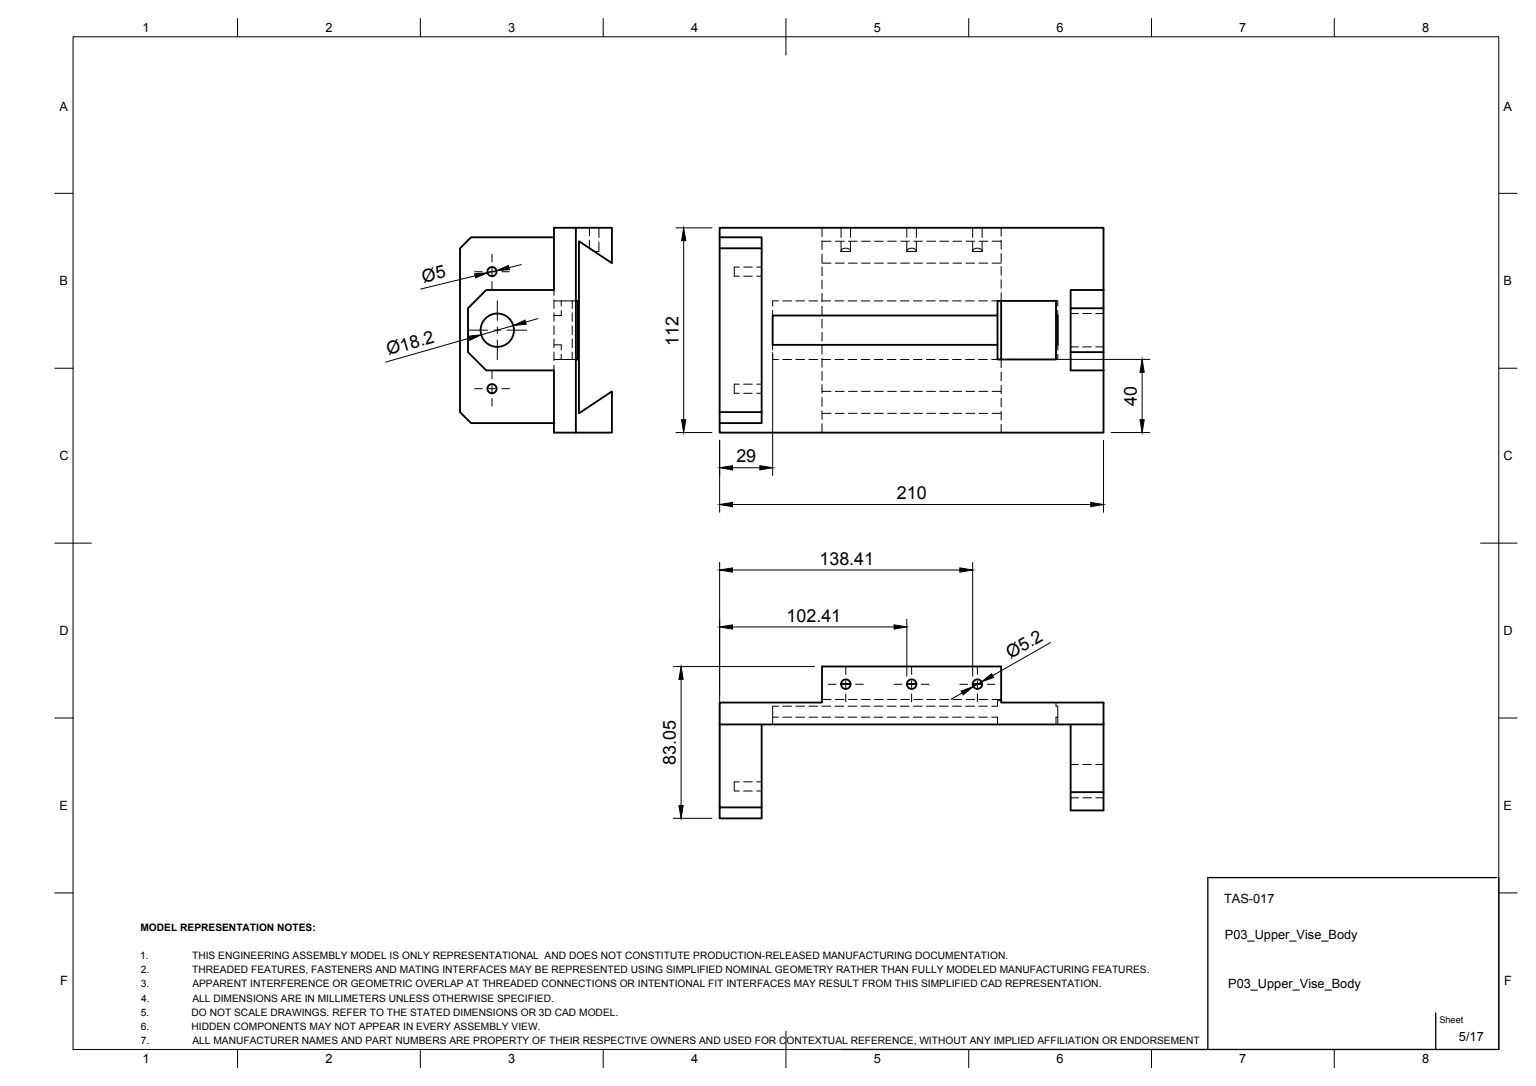
ISO-10303-21;
HEADER;
/* Generated by software containing ST-Developer
 * from STEP Tools, Inc. (www.steptools.com) 
 */

FILE_DESCRIPTION(
/* description */ ('STEP AP203'),
/* implementation_level */ '2;1');

FILE_NAME(
/* name */ 'P03_Upper_Vise_Body.step',
/* time_stamp */ '2026-11-15T15:04:01-08:00',
/* author */ (''),
/* organization */ (''),
/* preprocessor_version */ 'ST-DEVELOPER v20.2',
/* originating_system */ 'Autodesk Translation Framework v15.17.0.0',
/* authorisation */ '');

FILE_SCHEMA (('AUTOMOTIVE_DESIGN { 1 0 10303 214 3 1 1 }'));
ENDSEC;

DATA;
#10=MECHANICAL_DESIGN_GEOMETRIC_PRESENTATION_REPRESENTATION('',(#282),#16598);
#201=ELLIPSE('',#10193,3.12481110540202,2.59999999999971);
#202=ELLIPSE('',#10198,3.1248111054012,2.59999999999909);
#203=ELLIPSE('',#10203,3.12481110540162,2.59999999999945);
#206=SHAPE_REPRESENTATION_RELATIONSHIP('SRR','None',#16700,#230);
#230=ADVANCED_BREP_SHAPE_REPRESENTATION('',(#254),#16576);
#254=MANIFOLD_SOLID_BREP('Body1',#9789);
#282=STYLED_ITEM('',(#16830),#254);
#320=FACE_BOUND('',#1569,.T.);
#321=FACE_BOUND('',#1583,.T.);
#322=FACE_BOUND('',#1584,.T.);
#323=FACE_BOUND('',#1585,.T.);
#324=FACE_BOUND('',#1587,.T.);
#325=FACE_BOUND('',#1588,.T.);
#326=FACE_BOUND('',#1589,.T.);
#327=FACE_BOUND('',#1597,.T.);
#328=FACE_BOUND('',#1606,.T.);
#329=FACE_BOUND('',#1607,.T.);
#330=FACE_BOUND('',#1614,.T.);
#506=PLANE('',#10214);
#507=PLANE('',#10215);
#508=PLANE('',#10216);
#509=PLANE('',#10217);
#510=PLANE('',#10218);
#511=PLANE('',#10219);
#512=PLANE('',#10220);
#513=PLANE('',#10221);
#514=PLANE('',#10222);
#515=PLANE('',#10223);
#516=PLANE('',#10224);
#517=PLANE('',#10225);
#518=PLANE('',#10226);
#519=PLANE('',#10227);
#520=PLANE('',#10228);
#521=PLANE('',#10229);
#522=PLANE('',#10230);
#523=PLANE('',#10231);
#524=PLANE('',#10232);
#525=PLANE('',#10233);
#526=PLANE('',#10234);
#527=PLANE('',#10235);
#528=PLANE('',#10236);
#529=PLANE('',#10237);
#530=PLANE('',#10238);
#531=PLANE('',#10239);
#532=PLANE('',#10240);
#533=PLANE('',#10241);
#534=PLANE('',#10242);
#535=PLANE('',#10243);
#536=PLANE('',#10244);
#537=PLANE('',#10245);
#538=PLANE('',#10246);
#539=PLANE('',#10247);
#540=PLANE('',#10248);
#541=PLANE('',#10249);
#542=PLANE('',#10250);
#543=PLANE('',#10251);
#544=PLANE('',#10252);
#545=PLANE('',#10253);
#546=PLANE('',#10254);
#547=PLANE('',#10255);
#548=PLANE('',#10256);
#549=PLANE('',#10257);
#550=PLANE('',#10258);
#551=PLANE('',#10259);
#552=PLANE('',#10260);
#553=PLANE('',#10261);
#554=PLANE('',#10262);
#555=PLANE('',#10263);
#556=PLANE('',#10264);
#557=PLANE('',#10265);
#997=FACE_OUTER_BOUND('',#1562,.T.);
#998=FACE_OUTER_BOUND('',#1563,.T.);
#999=FACE_OUTER_BOUND('',#1564,.T.);
#1000=FACE_OUTER_BOUND('',#1565,.T.);
#1001=FACE_OUTER_BOUND('',#1566,.T.);
#1002=FACE_OUTER_BOUND('',#1567,.T.);
#1003=FACE_OUTER_BOUND('',#1568,.T.);
#1004=FACE_OUTER_BOUND('',#1570,.T.);
#1005=FACE_OUTER_BOUND('',#1571,.T.);
#1006=FACE_OUTER_BOUND('',#1572,.T.);
#1007=FACE_OUTER_BOUND('',#1573,.T.);
#1008=FACE_OUTER_BOUND('',#1574,.T.);
#1009=FACE_OUTER_BOUND('',#1575,.T.);
#1010=FACE_OUTER_BOUND('',#1576,.T.);
#1011=FACE_OUTER_BOUND('',#1577,.T.);
#1012=FACE_OUTER_BOUND('',#1578,.T.);
#1013=FACE_OUTER_BOUND('',#1579,.T.);
#1014=FACE_OUTER_BOUND('',#1580,.T.);
#1015=FACE_OUTER_BOUND('',#1581,.T.);
#1016=FACE_OUTER_BOUND('',#1582,.T.);
#1017=FACE_OUTER_BOUND('',#1586,.T.);
#1018=FACE_OUTER_BOUND('',#1590,.T.);
#1019=FACE_OUTER_BOUND('',#1591,.T.);
#1020=FACE_OUTER_BOUND('',#1592,.T.);
#1021=FACE_OUTER_BOUND('',#1593,.T.);
#1022=FACE_OUTER_BOUND('',#1594,.T.);
#1023=FACE_OUTER_BOUND('',#1595,.T.);
#1024=FACE_OUTER_BOUND('',#1596,.T.);
#1025=FACE_OUTER_BOUND('',#1598,.T.);
#1026=FACE_OUTER_BOUND('',#1599,.T.);
#1027=FACE_OUTER_BOUND('',#1600,.T.);
#1028=FACE_OUTER_BOUND('',#1601,.T.);
#1029=FACE_OUTER_BOUND('',#1602,.T.);
#1030=FACE_OUTER_BOUND('',#1603,.T.);
#1031=FACE_OUTER_BOUND('',#1604,.T.);
#1032=FACE_OUTER_BOUND('',#1605,.T.);
#1033=FACE_OUTER_BOUND('',#1608,.T.);
#1034=FACE_OUTER_BOUND('',#1609,.T.);
#1035=FACE_OUTER_BOUND('',#1610,.T.);
#1036=FACE_OUTER_BOUND('',#1611,.T.);
#1037=FACE_OUTER_BOUND('',#1612,.T.);
#1038=FACE_OUTER_BOUND('',#1613,.T.);
#1039=FACE_OUTER_BOUND('',#1615,.T.);
#1040=FACE_OUTER_BOUND('',#1616,.T.);
#1041=FACE_OUTER_BOUND('',#1617,.T.);
#1042=FACE_OUTER_BOUND('',#1618,.T.);
#1043=FACE_OUTER_BOUND('',#1619,.T.);
#1044=FACE_OUTER_BOUND('',#1620,.T.);
#1045=FACE_OUTER_BOUND('',#1621,.T.);
#1046=FACE_OUTER_BOUND('',#1622,.T.);
#1047=FACE_OUTER_BOUND('',#1623,.T.);
#1048=FACE_OUTER_BOUND('',#1624,.T.);
#1049=FACE_OUTER_BOUND('',#1625,.T.);
#1050=FACE_OUTER_BOUND('',#1626,.T.);
#1051=FACE_OUTER_BOUND('',#1627,.T.);
#1052=FACE_OUTER_BOUND('',#1628,.T.);
#1053=FACE_OUTER_BOUND('',#1629,.T.);
#1054=FACE_OUTER_BOUND('',#1630,.T.);
#1562=EDGE_LOOP('',(#7041,#7042,#7043,#7044,#7045,#7046));
#1563=EDGE_LOOP('',(#7047,#7048,#7049,#7050,#7051,#7052));
#1564=EDGE_LOOP('',(#7053,#7054,#7055,#7056,#7057,#7058));
#1565=EDGE_LOOP('',(#7059,#7060,#7061,#7062));
#1566=EDGE_LOOP('',(#7063,#7064,#7065,#7066));
#1567=EDGE_LOOP('',(#7067,#7068,#7069,#7070));
#1568=EDGE_LOOP('',(#7071,#7072,#7073,#7074,#7075,#7076,#7077,#7078,#7079,
#7080,#7081,#7082));
#1569=EDGE_LOOP('',(#7083,#7084,#7085,#7086,#7087,#7088,#7089,#7090,#7091,
#7092,#7093,#7094));
#1570=EDGE_LOOP('',(#7095,#7096,#7097,#7098,#7099,#7100,#7101,#7102,#7103,
#7104,#7105,#7106));
#1571=EDGE_LOOP('',(#7107,#7108,#7109,#7110,#7111,#7112,#7113,#7114));
#1572=EDGE_LOOP('',(#7115,#7116,#7117,#7118));
#1573=EDGE_LOOP('',(#7119,#7120,#7121,#7122));
#1574=EDGE_LOOP('',(#7123,#7124,#7125,#7126));
#1575=EDGE_LOOP('',(#7127,#7128,#7129,#7130));
#1576=EDGE_LOOP('',(#7131,#7132,#7133,#7134));
#1577=EDGE_LOOP('',(#7135,#7136,#7137,#7138));
#1578=EDGE_LOOP('',(#7139,#7140,#7141,#7142));
#1579=EDGE_LOOP('',(#7143,#7144,#7145,#7146));
#1580=EDGE_LOOP('',(#7147,#7148,#7149,#7150));
#1581=EDGE_LOOP('',(#7151,#7152,#7153,#7154));
#1582=EDGE_LOOP('',(#7155,#7156,#7157,#7158));
#1583=EDGE_LOOP('',(#7159,#7160));
#1584=EDGE_LOOP('',(#7161,#7162));
#1585=EDGE_LOOP('',(#7163,#7164));
#1586=EDGE_LOOP('',(#7165,#7166,#7167,#7168,#7169,#7170,#7171,#7172));
#1587=EDGE_LOOP('',(#7173));
#1588=EDGE_LOOP('',(#7174));
#1589=EDGE_LOOP('',(#7175));
#1590=EDGE_LOOP('',(#7176,#7177,#7178,#7179));
#1591=EDGE_LOOP('',(#7180,#7181,#7182,#7183));
#1592=EDGE_LOOP('',(#7184,#7185,#7186,#7187));
#1593=EDGE_LOOP('',(#7188,#7189,#7190,#7191));
#1594=EDGE_LOOP('',(#7192,#7193,#7194,#7195,#7196,#7197,#7198,#7199));
#1595=EDGE_LOOP('',(#7200,#7201,#7202,#7203,#7204,#7205,#7206,#7207));
#1596=EDGE_LOOP('',(#7208,#7209,#7210,#7211,#7212,#7213,#7214,#7215,#7216,
#7217));
#1597=EDGE_LOOP('',(#7218));
#1598=EDGE_LOOP('',(#7219,#7220,#7221,#7222));
#1599=EDGE_LOOP('',(#7223,#7224,#7225,#7226,#7227,#7228,#7229,#7230,#7231,
#7232));
#1600=EDGE_LOOP('',(#7233,#7234,#7235,#7236));
#1601=EDGE_LOOP('',(#7237,#7238,#7239,#7240));
#1602=EDGE_LOOP('',(#7241,#7242,#7243,#7244));
#1603=EDGE_LOOP('',(#7245,#7246,#7247,#7248));
#1604=EDGE_LOOP('',(#7249,#7250,#7251,#7252));
#1605=EDGE_LOOP('',(#7253,#7254,#7255,#7256,#7257,#7258));
#1606=EDGE_LOOP('',(#7259));
#1607=EDGE_LOOP('',(#7260));
#1608=EDGE_LOOP('',(#7261,#7262,#7263,#7264));
#1609=EDGE_LOOP('',(#7265,#7266,#7267,#7268));
#1610=EDGE_LOOP('',(#7269,#7270,#7271,#7272));
#1611=EDGE_LOOP('',(#7273,#7274,#7275,#7276));
#1612=EDGE_LOOP('',(#7277,#7278,#7279,#7280));
#1613=EDGE_LOOP('',(#7281,#7282,#7283,#7284,#7285,#7286));
#1614=EDGE_LOOP('',(#7287));
#1615=EDGE_LOOP('',(#7288,#7289,#7290,#7291,#7292,#7293,#7294,#7295));
#1616=EDGE_LOOP('',(#7296,#7297,#7298,#7299,#7300,#7301,#7302,#7303));
#1617=EDGE_LOOP('',(#7304,#7305,#7306,#7307,#7308,#7309,#7310,#7311,#7312,
#7313,#7314,#7315,#7316,#7317));
#1618=EDGE_LOOP('',(#7318,#7319,#7320,#7321,#7322,#7323,#7324,#7325,#7326,
#7327,#7328,#7329,#7330,#7331));
#1619=EDGE_LOOP('',(#7332));
#1620=EDGE_LOOP('',(#7333));
#1621=EDGE_LOOP('',(#7334,#7335,#7336));
#1622=EDGE_LOOP('',(#7337,#7338,#7339));
#1623=EDGE_LOOP('',(#7340,#7341,#7342));
#1624=EDGE_LOOP('',(#7343,#7344,#7345,#7346));
#1625=EDGE_LOOP('',(#7347,#7348,#7349,#7350));
#1626=EDGE_LOOP('',(#7351,#7352,#7353,#7354));
#1627=EDGE_LOOP('',(#7355,#7356,#7357,#7358));
#1628=EDGE_LOOP('',(#7359,#7360,#7361,#7362));
#1629=EDGE_LOOP('',(#7363,#7364,#7365,#7366));
#1630=EDGE_LOOP('',(#7367,#7368,#7369,#7370));
#2334=LINE('',#14144,#3382);
#2335=LINE('',#14154,#3383);
#2336=LINE('',#14164,#3384);
#2337=LINE('',#14174,#3385);
#2338=LINE('',#14180,#3386);
#2339=LINE('',#14186,#3387);
#2340=LINE('',#14191,#3388);
#2341=LINE('',#14193,#3389);
#2342=LINE('',#14195,#3390);
#2343=LINE('',#14197,#3391);
#2344=LINE('',#14199,#3392);
#2345=LINE('',#14201,#3393);
#2346=LINE('',#14203,#3394);
#2347=LINE('',#14205,#3395);
#2348=LINE('',#14207,#3396);
#2349=LINE('',#14209,#3397);
#2350=LINE('',#14211,#3398);
#2351=LINE('',#14212,#3399);
#2352=LINE('',#14215,#3400);
#2353=LINE('',#14217,#3401);
#2354=LINE('',#14219,#3402);
#2355=LINE('',#14221,#3403);
#2356=LINE('',#14223,#3404);
#2357=LINE('',#14225,#3405);
#2358=LINE('',#14227,#3406);
#2359=LINE('',#14229,#3407);
#2360=LINE('',#14231,#3408);
#2361=LINE('',#14233,#3409);
#2362=LINE('',#14235,#3410);
#2363=LINE('',#14236,#3411);
#2364=LINE('',#14240,#3412);
#2365=LINE('',#14242,#3413);
#2366=LINE('',#14244,#3414);
#2367=LINE('',#14246,#3415);
#2368=LINE('',#14248,#3416);
#2369=LINE('',#14250,#3417);
#2370=LINE('',#14252,#3418);
#2371=LINE('',#14254,#3419);
#2372=LINE('',#14256,#3420);
#2373=LINE('',#14258,#3421);
#2374=LINE('',#14260,#3422);
#2375=LINE('',#14261,#3423);
#2376=LINE('',#14264,#3424);
#2377=LINE('',#14266,#3425);
#2378=LINE('',#14267,#3426);
#2379=LINE('',#14269,#3427);
#2380=LINE('',#14271,#3428);
#2381=LINE('',#14272,#3429);
#2382=LINE('',#14275,#3430);
#2383=LINE('',#14277,#3431);
#2384=LINE('',#14278,#3432);
#2385=LINE('',#14282,#3433);
#2386=LINE('',#14283,#3434);
#2387=LINE('',#14284,#3435);
#2388=LINE('',#14288,#3436);
#2389=LINE('',#14289,#3437);
#2390=LINE('',#14290,#3438);
#2391=LINE('',#14293,#3439);
#2392=LINE('',#14295,#3440);
#2393=LINE('',#14296,#3441);
#2394=LINE('',#14299,#3442);
#2395=LINE('',#14301,#3443);
#2396=LINE('',#14302,#3444);
#2397=LINE('',#14306,#3445);
#2398=LINE('',#14307,#3446);
#2399=LINE('',#14308,#3447);
#2400=LINE('',#14312,#3448);
#2401=LINE('',#14314,#3449);
#2402=LINE('',#14316,#3450);
#2403=LINE('',#14317,#3451);
#2404=LINE('',#14321,#3452);
#2405=LINE('',#14323,#3453);
#2406=LINE('',#14325,#3454);
#2407=LINE('',#14326,#3455);
#2408=LINE('',#14330,#3456);
#2409=LINE('',#14331,#3457);
#2410=LINE('',#14332,#3458);
#2411=LINE('',#14335,#3459);
#2412=LINE('',#14337,#3460);
#2413=LINE('',#14338,#3461);
#2414=LINE('',#14341,#3462);
#2415=LINE('',#14343,#3463);
#2416=LINE('',#14344,#3464);
#2417=LINE('',#14345,#3465);
#2418=LINE('',#14346,#3466);
#2419=LINE('',#14347,#3467);
#2420=LINE('',#14351,#3468);
#2421=LINE('',#14353,#3469);
#2422=LINE('',#14354,#3470);
#2423=LINE('',#14355,#3471);
#2424=LINE('',#14356,#3472);
#2425=LINE('',#14358,#3473);
#2426=LINE('',#14361,#3474);
#2427=LINE('',#14362,#3475);
#2428=LINE('',#14365,#3476);
#2429=LINE('',#14366,#3477);
#2430=LINE('',#14369,#3478);
#2431=LINE('',#14370,#3479);
#2432=LINE('',#14372,#3480);
#2433=LINE('',#14374,#3481);
#2434=LINE('',#14376,#3482);
#2435=LINE('',#14377,#3483);
#2436=LINE('',#14379,#3484);
#2437=LINE('',#14382,#3485);
#2438=LINE('',#14384,#3486);
#2439=LINE('',#14386,#3487);
#2440=LINE('',#14388,#3488);
#2441=LINE('',#14389,#3489);
#2442=LINE('',#14391,#3490);
#2443=LINE('',#14394,#3491);
#2444=LINE('',#14396,#3492);
#2445=LINE('',#14398,#3493);
#2446=LINE('',#14400,#3494);
#2447=LINE('',#14401,#3495);
#2448=LINE('',#14404,#3496);
#2449=LINE('',#14405,#3497);
#2450=LINE('',#14408,#3498);
#2451=LINE('',#14409,#3499);
#2452=LINE('',#14412,#3500);
#2453=LINE('',#14413,#3501);
#2454=LINE('',#14416,#3502);
#2455=LINE('',#14417,#3503);
#2456=LINE('',#14419,#3504);
#2457=LINE('',#14423,#3505);
#2458=LINE('',#14424,#3506);
#2459=LINE('',#14427,#3507);
#2460=LINE('',#14428,#3508);
#2461=LINE('',#14431,#3509);
#2462=LINE('',#14432,#3510);
#2463=LINE('',#14435,#3511);
#2464=LINE('',#14436,#3512);
#2465=LINE('',#14438,#3513);
#2466=LINE('',#14441,#3514);
#2467=LINE('',#14442,#3515);
#2468=LINE('',#14444,#3516);
#2469=LINE('',#14445,#3517);
#2470=LINE('',#14447,#3518);
#2471=LINE('',#14448,#3519);
#2472=LINE('',#14449,#3520);
#2473=LINE('',#14451,#3521);
#2474=LINE('',#14452,#3522);
#2475=LINE('',#14454,#3523);
#2476=LINE('',#14455,#3524);
#2477=LINE('',#14457,#3525);
#2478=LINE('',#14458,#3526);
#2479=LINE('',#14459,#3527);
#2480=LINE('',#14468,#3528);
#3382=VECTOR('',#11358,2.59999999999999);
#3383=VECTOR('',#11369,2.59999999999999);
#3384=VECTOR('',#11380,2.59999999999999);
#3385=VECTOR('',#11391,2.5);
#3386=VECTOR('',#11398,2.5);
#3387=VECTOR('',#11405,9.1);
#3388=VECTOR('',#11410,1000.);
#3389=VECTOR('',#11411,1000.);
#3390=VECTOR('',#11412,1000.);
#3391=VECTOR('',#11413,1000.);
#3392=VECTOR('',#11414,1000.);
#3393=VECTOR('',#11415,1000.);
#3394=VECTOR('',#11416,1000.);
#3395=VECTOR('',#11417,1000.);
#3396=VECTOR('',#11418,1000.);
#3397=VECTOR('',#11419,1000.);
#3398=VECTOR('',#11420,1000.);
#3399=VECTOR('',#11421,1000.);
#3400=VECTOR('',#11422,1000.);
#3401=VECTOR('',#11423,1000.);
#3402=VECTOR('',#11424,1000.);
#3403=VECTOR('',#11425,1000.);
#3404=VECTOR('',#11426,1000.);
#3405=VECTOR('',#11427,1000.);
#3406=VECTOR('',#11428,1000.);
#3407=VECTOR('',#11429,1000.);
#3408=VECTOR('',#11430,1000.);
#3409=VECTOR('',#11431,1000.);
#3410=VECTOR('',#11432,1000.);
#3411=VECTOR('',#11433,1000.);
#3412=VECTOR('',#11436,1000.);
#3413=VECTOR('',#11437,1000.);
#3414=VECTOR('',#11438,1000.);
#3415=VECTOR('',#11439,1000.);
#3416=VECTOR('',#11440,1000.);
#3417=VECTOR('',#11441,1000.);
#3418=VECTOR('',#11442,1000.);
#3419=VECTOR('',#11443,1000.);
#3420=VECTOR('',#11444,1000.);
#3421=VECTOR('',#11445,1000.);
#3422=VECTOR('',#11446,1000.);
#3423=VECTOR('',#11447,1000.);
#3424=VECTOR('',#11450,1000.);
#3425=VECTOR('',#11451,1000.);
#3426=VECTOR('',#11452,1000.);
#3427=VECTOR('',#11453,1000.);
#3428=VECTOR('',#11454,1000.);
#3429=VECTOR('',#11455,1000.);
#3430=VECTOR('',#11458,1000.);
#3431=VECTOR('',#11459,1000.);
#3432=VECTOR('',#11460,1000.);
#3433=VECTOR('',#11463,1000.);
#3434=VECTOR('',#11464,1000.);
#3435=VECTOR('',#11465,1000.);
#3436=VECTOR('',#11468,1000.);
#3437=VECTOR('',#11469,1000.);
#3438=VECTOR('',#11470,1000.);
#3439=VECTOR('',#11473,1000.);
#3440=VECTOR('',#11474,1000.);
#3441=VECTOR('',#11475,1000.);
#3442=VECTOR('',#11478,1000.);
#3443=VECTOR('',#11479,1000.);
#3444=VECTOR('',#11480,1000.);
#3445=VECTOR('',#11483,1000.);
#3446=VECTOR('',#11484,1000.);
#3447=VECTOR('',#11485,1000.);
#3448=VECTOR('',#11488,1000.);
#3449=VECTOR('',#11489,1000.);
#3450=VECTOR('',#11490,1000.);
#3451=VECTOR('',#11491,1000.);
#3452=VECTOR('',#11494,1000.);
#3453=VECTOR('',#11495,1000.);
#3454=VECTOR('',#11496,1000.);
#3455=VECTOR('',#11497,1000.);
#3456=VECTOR('',#11500,1000.);
#3457=VECTOR('',#11501,1000.);
#3458=VECTOR('',#11502,1000.);
#3459=VECTOR('',#11505,1000.);
#3460=VECTOR('',#11506,1000.);
#3461=VECTOR('',#11507,1000.);
#3462=VECTOR('',#11510,1000.);
#3463=VECTOR('',#11511,1000.);
#3464=VECTOR('',#11512,1000.);
#3465=VECTOR('',#11513,1000.);
#3466=VECTOR('',#11514,1000.);
#3467=VECTOR('',#11515,1000.);
#3468=VECTOR('',#11518,1000.);
#3469=VECTOR('',#11519,1000.);
#3470=VECTOR('',#11520,1000.);
#3471=VECTOR('',#11521,1000.);
#3472=VECTOR('',#11522,1000.);
#3473=VECTOR('',#11525,1000.);
#3474=VECTOR('',#11528,1000.);
#3475=VECTOR('',#11529,1000.);
#3476=VECTOR('',#11532,1000.);
#3477=VECTOR('',#11533,1000.);
#3478=VECTOR('',#11536,1000.);
#3479=VECTOR('',#11537,1000.);
#3480=VECTOR('',#11540,1000.);
#3481=VECTOR('',#11541,1000.);
#3482=VECTOR('',#11542,1000.);
#3483=VECTOR('',#11543,1000.);
#3484=VECTOR('',#11546,1000.);
#3485=VECTOR('',#11549,1000.);
#3486=VECTOR('',#11550,1000.);
#3487=VECTOR('',#11551,1000.);
#3488=VECTOR('',#11552,1000.);
#3489=VECTOR('',#11553,1000.);
#3490=VECTOR('',#11556,1000.);
#3491=VECTOR('',#11559,1000.);
#3492=VECTOR('',#11560,1000.);
#3493=VECTOR('',#11561,1000.);
#3494=VECTOR('',#11562,1000.);
#3495=VECTOR('',#11563,1000.);
#3496=VECTOR('',#11566,1000.);
#3497=VECTOR('',#11567,1000.);
#3498=VECTOR('',#11570,1000.);
#3499=VECTOR('',#11571,1000.);
#3500=VECTOR('',#11574,1000.);
#3501=VECTOR('',#11575,1000.);
#3502=VECTOR('',#11578,1000.);
#3503=VECTOR('',#11579,1000.);
#3504=VECTOR('',#11582,1000.);
#3505=VECTOR('',#11587,1000.);
#3506=VECTOR('',#11588,1000.);
#3507=VECTOR('',#11591,1000.);
#3508=VECTOR('',#11592,1000.);
#3509=VECTOR('',#11595,1000.);
#3510=VECTOR('',#11596,1000.);
#3511=VECTOR('',#11599,1000.);
#3512=VECTOR('',#11600,1000.);
#3513=VECTOR('',#11603,1000.);
#3514=VECTOR('',#11608,1000.);
#3515=VECTOR('',#11609,1000.);
#3516=VECTOR('',#11612,1000.);
#3517=VECTOR('',#11613,1000.);
#3518=VECTOR('',#11616,1000.);
#3519=VECTOR('',#11617,1000.);
#3520=VECTOR('',#11618,1000.);
#3521=VECTOR('',#11619,1000.);
#3522=VECTOR('',#11620,1000.);
#3523=VECTOR('',#11623,1000.);
#3524=VECTOR('',#11624,1000.);
#3525=VECTOR('',#11625,1000.);
#3526=VECTOR('',#11626,1000.);
#3527=VECTOR('',#11627,1000.);
#3528=VECTOR('',#11644,1000.);
#4250=CIRCLE('',#10191,2.59999999999999);
#4251=CIRCLE('',#10192,2.6);
#4252=CIRCLE('',#10194,2.6);
#4253=CIRCLE('',#10196,2.59999999999999);
#4254=CIRCLE('',#10197,2.6);
#4255=CIRCLE('',#10199,2.6);
#4256=CIRCLE('',#10201,2.59999999999999);
#4257=CIRCLE('',#10202,2.6);
#4258=CIRCLE('',#10204,2.6);
#4259=CIRCLE('',#10206,2.5);
#4260=CIRCLE('',#10207,2.5);
#4261=CIRCLE('',#10209,2.5);
#4262=CIRCLE('',#10210,2.5);
#4263=CIRCLE('',#10212,9.1);
#4264=CIRCLE('',#10213,9.1);
#4603=VERTEX_POINT('',#14141);
#4604=VERTEX_POINT('',#14143);
#4605=VERTEX_POINT('',#14145);
#4606=VERTEX_POINT('',#14147);
#4607=VERTEX_POINT('',#14151);
#4608=VERTEX_POINT('',#14153);
#4609=VERTEX_POINT('',#14155);
#4610=VERTEX_POINT('',#14157);
#4611=VERTEX_POINT('',#14161);
#4612=VERTEX_POINT('',#14163);
#4613=VERTEX_POINT('',#14165);
#4614=VERTEX_POINT('',#14167);
#4615=VERTEX_POINT('',#14171);
#4616=VERTEX_POINT('',#14173);
#4617=VERTEX_POINT('',#14177);
#4618=VERTEX_POINT('',#14179);
#4619=VERTEX_POINT('',#14183);
#4620=VERTEX_POINT('',#14185);
#4621=VERTEX_POINT('',#14189);
#4622=VERTEX_POINT('',#14190);
#4623=VERTEX_POINT('',#14192);
#4624=VERTEX_POINT('',#14194);
#4625=VERTEX_POINT('',#14196);
#4626=VERTEX_POINT('',#14198);
#4627=VERTEX_POINT('',#14200);
#4628=VERTEX_POINT('',#14202);
#4629=VERTEX_POINT('',#14204);
#4630=VERTEX_POINT('',#14206);
#4631=VERTEX_POINT('',#14208);
#4632=VERTEX_POINT('',#14210);
#4633=VERTEX_POINT('',#14213);
#4634=VERTEX_POINT('',#14214);
#4635=VERTEX_POINT('',#14216);
#4636=VERTEX_POINT('',#14218);
#4637=VERTEX_POINT('',#14220);
#4638=VERTEX_POINT('',#14222);
#4639=VERTEX_POINT('',#14224);
#4640=VERTEX_POINT('',#14226);
#4641=VERTEX_POINT('',#14228);
#4642=VERTEX_POINT('',#14230);
#4643=VERTEX_POINT('',#14232);
#4644=VERTEX_POINT('',#14234);
#4645=VERTEX_POINT('',#14238);
#4646=VERTEX_POINT('',#14239);
#4647=VERTEX_POINT('',#14241);
#4648=VERTEX_POINT('',#14243);
#4649=VERTEX_POINT('',#14245);
#4650=VERTEX_POINT('',#14247);
#4651=VERTEX_POINT('',#14249);
#4652=VERTEX_POINT('',#14251);
#4653=VERTEX_POINT('',#14253);
#4654=VERTEX_POINT('',#14255);
#4655=VERTEX_POINT('',#14257);
#4656=VERTEX_POINT('',#14259);
#4657=VERTEX_POINT('',#14263);
#4658=VERTEX_POINT('',#14265);
#4659=VERTEX_POINT('',#14268);
#4660=VERTEX_POINT('',#14270);
#4661=VERTEX_POINT('',#14274);
#4662=VERTEX_POINT('',#14276);
#4663=VERTEX_POINT('',#14280);
#4664=VERTEX_POINT('',#14281);
#4665=VERTEX_POINT('',#14286);
#4666=VERTEX_POINT('',#14287);
#4667=VERTEX_POINT('',#14292);
#4668=VERTEX_POINT('',#14294);
#4669=VERTEX_POINT('',#14298);
#4670=VERTEX_POINT('',#14300);
#4671=VERTEX_POINT('',#14304);
#4672=VERTEX_POINT('',#14305);
#4673=VERTEX_POINT('',#14310);
#4674=VERTEX_POINT('',#14311);
#4675=VERTEX_POINT('',#14313);
#4676=VERTEX_POINT('',#14315);
#4677=VERTEX_POINT('',#14319);
#4678=VERTEX_POINT('',#14320);
#4679=VERTEX_POINT('',#14322);
#4680=VERTEX_POINT('',#14324);
#4681=VERTEX_POINT('',#14328);
#4682=VERTEX_POINT('',#14329);
#4683=VERTEX_POINT('',#14334);
#4684=VERTEX_POINT('',#14336);
#4685=VERTEX_POINT('',#14340);
#4686=VERTEX_POINT('',#14342);
#4687=VERTEX_POINT('',#14349);
#4688=VERTEX_POINT('',#14350);
#4689=VERTEX_POINT('',#14352);
#4690=VERTEX_POINT('',#14360);
#4691=VERTEX_POINT('',#14364);
#4692=VERTEX_POINT('',#14368);
#4693=VERTEX_POINT('',#14373);
#4694=VERTEX_POINT('',#14375);
#4695=VERTEX_POINT('',#14381);
#4696=VERTEX_POINT('',#14383);
#4697=VERTEX_POINT('',#14385);
#4698=VERTEX_POINT('',#14387);
#4699=VERTEX_POINT('',#14393);
#4700=VERTEX_POINT('',#14395);
#4701=VERTEX_POINT('',#14397);
#4702=VERTEX_POINT('',#14399);
#4703=VERTEX_POINT('',#14403);
#4704=VERTEX_POINT('',#14407);
#4705=VERTEX_POINT('',#14411);
#4706=VERTEX_POINT('',#14415);
#4707=VERTEX_POINT('',#14422);
#4708=VERTEX_POINT('',#14426);
#4709=VERTEX_POINT('',#14430);
#4710=VERTEX_POINT('',#14434);
#4711=VERTEX_POINT('',#14450);
#4712=VERTEX_POINT('',#14456);
#5533=EDGE_CURVE('',#4603,#4603,#4250,.T.);
#5534=EDGE_CURVE('',#4603,#4604,#2334,.T.);
#5535=EDGE_CURVE('',#4605,#4604,#4251,.T.);
#5536=EDGE_CURVE('',#4605,#4606,#201,.T.);
#5537=EDGE_CURVE('',#4604,#4606,#4252,.T.);
#5538=EDGE_CURVE('',#4607,#4607,#4253,.T.);
#5539=EDGE_CURVE('',#4607,#4608,#2335,.T.);
#5540=EDGE_CURVE('',#4609,#4608,#4254,.T.);
#5541=EDGE_CURVE('',#4609,#4610,#202,.T.);
#5542=EDGE_CURVE('',#4608,#4610,#4255,.T.);
#5543=EDGE_CURVE('',#4611,#4611,#4256,.T.);
#5544=EDGE_CURVE('',#4611,#4612,#2336,.T.);
#5545=EDGE_CURVE('',#4613,#4612,#4257,.T.);
#5546=EDGE_CURVE('',#4613,#4614,#203,.T.);
#5547=EDGE_CURVE('',#4612,#4614,#4258,.T.);
#5548=EDGE_CURVE('',#4615,#4615,#4259,.T.);
#5549=EDGE_CURVE('',#4615,#4616,#2337,.T.);
#5550=EDGE_CURVE('',#4616,#4616,#4260,.T.);
#5551=EDGE_CURVE('',#4617,#4617,#4261,.T.);
#5552=EDGE_CURVE('',#4617,#4618,#2338,.T.);
#5553=EDGE_CURVE('',#4618,#4618,#4262,.T.);
#5554=EDGE_CURVE('',#4619,#4619,#4263,.T.);
#5555=EDGE_CURVE('',#4619,#4620,#2339,.T.);
#5556=EDGE_CURVE('',#4620,#4620,#4264,.T.);
#5557=EDGE_CURVE('',#4621,#4622,#2340,.T.);
#5558=EDGE_CURVE('',#4623,#4621,#2341,.T.);
#5559=EDGE_CURVE('',#4623,#4624,#2342,.T.);
#5560=EDGE_CURVE('',#4624,#4625,#2343,.T.);
#5561=EDGE_CURVE('',#4626,#4625,#2344,.T.);
#5562=EDGE_CURVE('',#4626,#4627,#2345,.T.);
#5563=EDGE_CURVE('',#4627,#4628,#2346,.T.);
#5564=EDGE_CURVE('',#4628,#4629,#2347,.T.);
#5565=EDGE_CURVE('',#4630,#4629,#2348,.T.);
#5566=EDGE_CURVE('',#4630,#4631,#2349,.T.);
#5567=EDGE_CURVE('',#4631,#4632,#2350,.T.);
#5568=EDGE_CURVE('',#4632,#4622,#2351,.T.);
#5569=EDGE_CURVE('',#4633,#4634,#2352,.T.);
#5570=EDGE_CURVE('',#4635,#4633,#2353,.T.);
#5571=EDGE_CURVE('',#4635,#4636,#2354,.T.);
#5572=EDGE_CURVE('',#4637,#4636,#2355,.T.);
#5573=EDGE_CURVE('',#4638,#4637,#2356,.T.);
#5574=EDGE_CURVE('',#4639,#4638,#2357,.T.);
#5575=EDGE_CURVE('',#4640,#4639,#2358,.T.);
#5576=EDGE_CURVE('',#4641,#4640,#2359,.T.);
#5577=EDGE_CURVE('',#4642,#4641,#2360,.T.);
#5578=EDGE_CURVE('',#4643,#4642,#2361,.T.);
#5579=EDGE_CURVE('',#4644,#4643,#2362,.T.);
#5580=EDGE_CURVE('',#4634,#4644,#2363,.T.);
#5581=EDGE_CURVE('',#4645,#4646,#2364,.T.);
#5582=EDGE_CURVE('',#4646,#4647,#2365,.T.);
#5583=EDGE_CURVE('',#4648,#4647,#2366,.T.);
#5584=EDGE_CURVE('',#4649,#4648,#2367,.T.);
#5585=EDGE_CURVE('',#4650,#4649,#2368,.T.);
#5586=EDGE_CURVE('',#4651,#4650,#2369,.T.);
#5587=EDGE_CURVE('',#4652,#4651,#2370,.T.);
#5588=EDGE_CURVE('',#4653,#4652,#2371,.T.);
#5589=EDGE_CURVE('',#4654,#4653,#2372,.T.);
#5590=EDGE_CURVE('',#4655,#4654,#2373,.T.);
#5591=EDGE_CURVE('',#4656,#4655,#2374,.T.);
#5592=EDGE_CURVE('',#4656,#4645,#2375,.T.);
#5593=EDGE_CURVE('',#4647,#4657,#2376,.T.);
#5594=EDGE_CURVE('',#4657,#4658,#2377,.T.);
#5595=EDGE_CURVE('',#4658,#4656,#2378,.T.);
#5596=EDGE_CURVE('',#4659,#4655,#2379,.T.);
#5597=EDGE_CURVE('',#4660,#4659,#2380,.T.);
#5598=EDGE_CURVE('',#4648,#4660,#2381,.T.);
#5599=EDGE_CURVE('',#4633,#4661,#2382,.T.);
#5600=EDGE_CURVE('',#4661,#4662,#2383,.T.);
#5601=EDGE_CURVE('',#4635,#4662,#2384,.T.);
#5602=EDGE_CURVE('',#4663,#4664,#2385,.T.);
#5603=EDGE_CURVE('',#4664,#4643,#2386,.T.);
#5604=EDGE_CURVE('',#4642,#4663,#2387,.T.);
#5605=EDGE_CURVE('',#4665,#4666,#2388,.T.);
#5606=EDGE_CURVE('',#4665,#4637,#2389,.T.);
#5607=EDGE_CURVE('',#4666,#4636,#2390,.T.);
#5608=EDGE_CURVE('',#4640,#4667,#2391,.T.);
#5609=EDGE_CURVE('',#4668,#4667,#2392,.T.);
#5610=EDGE_CURVE('',#4668,#4641,#2393,.T.);
#5611=EDGE_CURVE('',#4661,#4669,#2394,.T.);
#5612=EDGE_CURVE('',#4669,#4670,#2395,.T.);
#5613=EDGE_CURVE('',#4662,#4670,#2396,.T.);
#5614=EDGE_CURVE('',#4671,#4672,#2397,.T.);
#5615=EDGE_CURVE('',#4672,#4664,#2398,.T.);
#5616=EDGE_CURVE('',#4663,#4671,#2399,.T.);
#5617=EDGE_CURVE('',#4673,#4674,#2400,.T.);
#5618=EDGE_CURVE('',#4673,#4675,#2401,.T.);
#5619=EDGE_CURVE('',#4675,#4676,#2402,.T.);
#5620=EDGE_CURVE('',#4674,#4676,#2403,.T.);
#5621=EDGE_CURVE('',#4677,#4678,#2404,.T.);
#5622=EDGE_CURVE('',#4678,#4679,#2405,.T.);
#5623=EDGE_CURVE('',#4680,#4679,#2406,.T.);
#5624=EDGE_CURVE('',#4680,#4677,#2407,.T.);
#5625=EDGE_CURVE('',#4681,#4682,#2408,.T.);
#5626=EDGE_CURVE('',#4681,#4665,#2409,.T.);
#5627=EDGE_CURVE('',#4682,#4666,#2410,.T.);
#5628=EDGE_CURVE('',#4667,#4683,#2411,.T.);
#5629=EDGE_CURVE('',#4684,#4683,#2412,.T.);
#5630=EDGE_CURVE('',#4684,#4668,#2413,.T.);
#5631=EDGE_CURVE('',#4685,#4652,#2414,.T.);
#5632=EDGE_CURVE('',#4686,#4685,#2415,.T.);
#5633=EDGE_CURVE('',#4686,#4653,#2416,.T.);
#5634=EDGE_CURVE('',#4614,#4613,#2417,.T.);
#5635=EDGE_CURVE('',#4606,#4605,#2418,.T.);
#5636=EDGE_CURVE('',#4610,#4609,#2419,.T.);
#5637=EDGE_CURVE('',#4687,#4688,#2420,.T.);
#5638=EDGE_CURVE('',#4687,#4689,#2421,.T.);
#5639=EDGE_CURVE('',#4626,#4689,#2422,.T.);
#5640=EDGE_CURVE('',#4625,#4659,#2423,.T.);
#5641=EDGE_CURVE('',#4688,#4654,#2424,.T.);
#5642=EDGE_CURVE('',#4688,#4686,#2425,.T.);
#5643=EDGE_CURVE('',#4690,#4651,#2426,.T.);
#5644=EDGE_CURVE('',#4685,#4690,#2427,.T.);
#5645=EDGE_CURVE('',#4691,#4650,#2428,.T.);
#5646=EDGE_CURVE('',#4690,#4691,#2429,.T.);
#5647=EDGE_CURVE('',#4692,#4649,#2430,.T.);
#5648=EDGE_CURVE('',#4691,#4692,#2431,.T.);
#5649=EDGE_CURVE('',#4632,#4660,#2432,.T.);
#5650=EDGE_CURVE('',#4631,#4693,#2433,.T.);
#5651=EDGE_CURVE('',#4693,#4694,#2434,.T.);
#5652=EDGE_CURVE('',#4692,#4694,#2435,.T.);
#5653=EDGE_CURVE('',#4694,#4687,#2436,.T.);
#5654=EDGE_CURVE('',#4695,#4624,#2437,.T.);
#5655=EDGE_CURVE('',#4696,#4695,#2438,.T.);
#5656=EDGE_CURVE('',#4697,#4696,#2439,.T.);
#5657=EDGE_CURVE('',#4698,#4697,#2440,.T.);
#5658=EDGE_CURVE('',#4622,#4698,#2441,.T.);
#5659=EDGE_CURVE('',#4689,#4693,#2442,.T.);
#5660=EDGE_CURVE('',#4630,#4699,#2443,.T.);
#5661=EDGE_CURVE('',#4699,#4700,#2444,.T.);
#5662=EDGE_CURVE('',#4700,#4701,#2445,.T.);
#5663=EDGE_CURVE('',#4701,#4702,#2446,.T.);
#5664=EDGE_CURVE('',#4702,#4627,#2447,.T.);
#5665=EDGE_CURVE('',#4629,#4703,#2448,.T.);
#5666=EDGE_CURVE('',#4699,#4703,#2449,.T.);
#5667=EDGE_CURVE('',#4703,#4704,#2450,.T.);
#5668=EDGE_CURVE('',#4700,#4704,#2451,.T.);
#5669=EDGE_CURVE('',#4704,#4705,#2452,.T.);
#5670=EDGE_CURVE('',#4701,#4705,#2453,.T.);
#5671=EDGE_CURVE('',#4705,#4706,#2454,.T.);
#5672=EDGE_CURVE('',#4702,#4706,#2455,.T.);
#5673=EDGE_CURVE('',#4706,#4628,#2456,.T.);
#5674=EDGE_CURVE('',#4707,#4698,#2457,.T.);
#5675=EDGE_CURVE('',#4621,#4707,#2458,.T.);
#5676=EDGE_CURVE('',#4708,#4697,#2459,.T.);
#5677=EDGE_CURVE('',#4707,#4708,#2460,.T.);
#5678=EDGE_CURVE('',#4709,#4696,#2461,.T.);
#5679=EDGE_CURVE('',#4708,#4709,#2462,.T.);
#5680=EDGE_CURVE('',#4710,#4695,#2463,.T.);
#5681=EDGE_CURVE('',#4709,#4710,#2464,.T.);
#5682=EDGE_CURVE('',#4710,#4623,#2465,.T.);
#5683=EDGE_CURVE('',#4677,#4684,#2466,.T.);
#5684=EDGE_CURVE('',#4671,#4680,#2467,.T.);
#5685=EDGE_CURVE('',#4670,#4674,#2468,.T.);
#5686=EDGE_CURVE('',#4676,#4682,#2469,.T.);
#5687=EDGE_CURVE('',#4673,#4658,#2470,.T.);
#5688=EDGE_CURVE('',#4634,#4669,#2471,.T.);
#5689=EDGE_CURVE('',#4644,#4672,#2472,.T.);
#5690=EDGE_CURVE('',#4679,#4711,#2473,.T.);
#5691=EDGE_CURVE('',#4645,#4711,#2474,.T.);
#5692=EDGE_CURVE('',#4638,#4681,#2475,.T.);
#5693=EDGE_CURVE('',#4675,#4657,#2476,.T.);
#5694=EDGE_CURVE('',#4712,#4646,#2477,.T.);
#5695=EDGE_CURVE('',#4678,#4712,#2478,.T.);
#5696=EDGE_CURVE('',#4639,#4683,#2479,.T.);
#5697=EDGE_CURVE('',#4711,#4712,#2480,.T.);
#7041=ORIENTED_EDGE('',*,*,#5533,.T.);
#7042=ORIENTED_EDGE('',*,*,#5534,.T.);
#7043=ORIENTED_EDGE('',*,*,#5535,.F.);
#7044=ORIENTED_EDGE('',*,*,#5536,.T.);
#7045=ORIENTED_EDGE('',*,*,#5537,.F.);
#7046=ORIENTED_EDGE('',*,*,#5534,.F.);
#7047=ORIENTED_EDGE('',*,*,#5538,.T.);
#7048=ORIENTED_EDGE('',*,*,#5539,.T.);
#7049=ORIENTED_EDGE('',*,*,#5540,.F.);
#7050=ORIENTED_EDGE('',*,*,#5541,.T.);
#7051=ORIENTED_EDGE('',*,*,#5542,.F.);
#7052=ORIENTED_EDGE('',*,*,#5539,.F.);
#7053=ORIENTED_EDGE('',*,*,#5543,.T.);
#7054=ORIENTED_EDGE('',*,*,#5544,.T.);
#7055=ORIENTED_EDGE('',*,*,#5545,.F.);
#7056=ORIENTED_EDGE('',*,*,#5546,.T.);
#7057=ORIENTED_EDGE('',*,*,#5547,.F.);
#7058=ORIENTED_EDGE('',*,*,#5544,.F.);
#7059=ORIENTED_EDGE('',*,*,#5548,.T.);
#7060=ORIENTED_EDGE('',*,*,#5549,.T.);
#7061=ORIENTED_EDGE('',*,*,#5550,.F.);
#7062=ORIENTED_EDGE('',*,*,#5549,.F.);
#7063=ORIENTED_EDGE('',*,*,#5551,.T.);
#7064=ORIENTED_EDGE('',*,*,#5552,.T.);
#7065=ORIENTED_EDGE('',*,*,#5553,.F.);
#7066=ORIENTED_EDGE('',*,*,#5552,.F.);
#7067=ORIENTED_EDGE('',*,*,#5554,.T.);
#7068=ORIENTED_EDGE('',*,*,#5555,.T.);
#7069=ORIENTED_EDGE('',*,*,#5556,.T.);
#7070=ORIENTED_EDGE('',*,*,#5555,.F.);
#7071=ORIENTED_EDGE('',*,*,#5557,.F.);
#7072=ORIENTED_EDGE('',*,*,#5558,.F.);
#7073=ORIENTED_EDGE('',*,*,#5559,.T.);
#7074=ORIENTED_EDGE('',*,*,#5560,.T.);
#7075=ORIENTED_EDGE('',*,*,#5561,.F.);
#7076=ORIENTED_EDGE('',*,*,#5562,.T.);
#7077=ORIENTED_EDGE('',*,*,#5563,.T.);
#7078=ORIENTED_EDGE('',*,*,#5564,.T.);
#7079=ORIENTED_EDGE('',*,*,#5565,.F.);
#7080=ORIENTED_EDGE('',*,*,#5566,.T.);
#7081=ORIENTED_EDGE('',*,*,#5567,.T.);
#7082=ORIENTED_EDGE('',*,*,#5568,.T.);
#7083=ORIENTED_EDGE('',*,*,#5569,.F.);
#7084=ORIENTED_EDGE('',*,*,#5570,.F.);
#7085=ORIENTED_EDGE('',*,*,#5571,.T.);
#7086=ORIENTED_EDGE('',*,*,#5572,.F.);
#7087=ORIENTED_EDGE('',*,*,#5573,.F.);
#7088=ORIENTED_EDGE('',*,*,#5574,.F.);
#7089=ORIENTED_EDGE('',*,*,#5575,.F.);
#7090=ORIENTED_EDGE('',*,*,#5576,.F.);
#7091=ORIENTED_EDGE('',*,*,#5577,.F.);
#7092=ORIENTED_EDGE('',*,*,#5578,.F.);
#7093=ORIENTED_EDGE('',*,*,#5579,.F.);
#7094=ORIENTED_EDGE('',*,*,#5580,.F.);
#7095=ORIENTED_EDGE('',*,*,#5581,.T.);
#7096=ORIENTED_EDGE('',*,*,#5582,.T.);
#7097=ORIENTED_EDGE('',*,*,#5583,.F.);
#7098=ORIENTED_EDGE('',*,*,#5584,.F.);
#7099=ORIENTED_EDGE('',*,*,#5585,.F.);
#7100=ORIENTED_EDGE('',*,*,#5586,.F.);
#7101=ORIENTED_EDGE('',*,*,#5587,.F.);
#7102=ORIENTED_EDGE('',*,*,#5588,.F.);
#7103=ORIENTED_EDGE('',*,*,#5589,.F.);
#7104=ORIENTED_EDGE('',*,*,#5590,.F.);
#7105=ORIENTED_EDGE('',*,*,#5591,.F.);
#7106=ORIENTED_EDGE('',*,*,#5592,.T.);
#7107=ORIENTED_EDGE('',*,*,#5583,.T.);
#7108=ORIENTED_EDGE('',*,*,#5593,.T.);
#7109=ORIENTED_EDGE('',*,*,#5594,.T.);
#7110=ORIENTED_EDGE('',*,*,#5595,.T.);
#7111=ORIENTED_EDGE('',*,*,#5591,.T.);
#7112=ORIENTED_EDGE('',*,*,#5596,.F.);
#7113=ORIENTED_EDGE('',*,*,#5597,.F.);
#7114=ORIENTED_EDGE('',*,*,#5598,.F.);
#7115=ORIENTED_EDGE('',*,*,#5570,.T.);
#7116=ORIENTED_EDGE('',*,*,#5599,.T.);
#7117=ORIENTED_EDGE('',*,*,#5600,.T.);
#7118=ORIENTED_EDGE('',*,*,#5601,.F.);
#7119=ORIENTED_EDGE('',*,*,#5602,.T.);
#7120=ORIENTED_EDGE('',*,*,#5603,.T.);
#7121=ORIENTED_EDGE('',*,*,#5578,.T.);
#7122=ORIENTED_EDGE('',*,*,#5604,.T.);
#7123=ORIENTED_EDGE('',*,*,#5605,.F.);
#7124=ORIENTED_EDGE('',*,*,#5606,.T.);
#7125=ORIENTED_EDGE('',*,*,#5572,.T.);
#7126=ORIENTED_EDGE('',*,*,#5607,.F.);
#7127=ORIENTED_EDGE('',*,*,#5576,.T.);
#7128=ORIENTED_EDGE('',*,*,#5608,.T.);
#7129=ORIENTED_EDGE('',*,*,#5609,.F.);
#7130=ORIENTED_EDGE('',*,*,#5610,.T.);
#7131=ORIENTED_EDGE('',*,*,#5600,.F.);
#7132=ORIENTED_EDGE('',*,*,#5611,.T.);
#7133=ORIENTED_EDGE('',*,*,#5612,.T.);
#7134=ORIENTED_EDGE('',*,*,#5613,.F.);
#7135=ORIENTED_EDGE('',*,*,#5614,.T.);
#7136=ORIENTED_EDGE('',*,*,#5615,.T.);
#7137=ORIENTED_EDGE('',*,*,#5602,.F.);
#7138=ORIENTED_EDGE('',*,*,#5616,.T.);
#7139=ORIENTED_EDGE('',*,*,#5617,.F.);
#7140=ORIENTED_EDGE('',*,*,#5618,.T.);
#7141=ORIENTED_EDGE('',*,*,#5619,.T.);
#7142=ORIENTED_EDGE('',*,*,#5620,.F.);
#7143=ORIENTED_EDGE('',*,*,#5621,.T.);
#7144=ORIENTED_EDGE('',*,*,#5622,.T.);
#7145=ORIENTED_EDGE('',*,*,#5623,.F.);
#7146=ORIENTED_EDGE('',*,*,#5624,.T.);
#7147=ORIENTED_EDGE('',*,*,#5625,.F.);
#7148=ORIENTED_EDGE('',*,*,#5626,.T.);
#7149=ORIENTED_EDGE('',*,*,#5605,.T.);
#7150=ORIENTED_EDGE('',*,*,#5627,.F.);
#7151=ORIENTED_EDGE('',*,*,#5609,.T.);
#7152=ORIENTED_EDGE('',*,*,#5628,.T.);
#7153=ORIENTED_EDGE('',*,*,#5629,.F.);
#7154=ORIENTED_EDGE('',*,*,#5630,.T.);
#7155=ORIENTED_EDGE('',*,*,#5588,.T.);
#7156=ORIENTED_EDGE('',*,*,#5631,.F.);
#7157=ORIENTED_EDGE('',*,*,#5632,.F.);
#7158=ORIENTED_EDGE('',*,*,#5633,.T.);
#7159=ORIENTED_EDGE('',*,*,#5546,.F.);
#7160=ORIENTED_EDGE('',*,*,#5634,.F.);
#7161=ORIENTED_EDGE('',*,*,#5536,.F.);
#7162=ORIENTED_EDGE('',*,*,#5635,.F.);
#7163=ORIENTED_EDGE('',*,*,#5541,.F.);
#7164=ORIENTED_EDGE('',*,*,#5636,.F.);
#7165=ORIENTED_EDGE('',*,*,#5637,.F.);
#7166=ORIENTED_EDGE('',*,*,#5638,.T.);
#7167=ORIENTED_EDGE('',*,*,#5639,.F.);
#7168=ORIENTED_EDGE('',*,*,#5561,.T.);
#7169=ORIENTED_EDGE('',*,*,#5640,.T.);
#7170=ORIENTED_EDGE('',*,*,#5596,.T.);
#7171=ORIENTED_EDGE('',*,*,#5590,.T.);
#7172=ORIENTED_EDGE('',*,*,#5641,.F.);
#7173=ORIENTED_EDGE('',*,*,#5533,.F.);
#7174=ORIENTED_EDGE('',*,*,#5538,.F.);
#7175=ORIENTED_EDGE('',*,*,#5543,.F.);
#7176=ORIENTED_EDGE('',*,*,#5589,.T.);
#7177=ORIENTED_EDGE('',*,*,#5633,.F.);
#7178=ORIENTED_EDGE('',*,*,#5642,.F.);
#7179=ORIENTED_EDGE('',*,*,#5641,.T.);
#7180=ORIENTED_EDGE('',*,*,#5587,.T.);
#7181=ORIENTED_EDGE('',*,*,#5643,.F.);
#7182=ORIENTED_EDGE('',*,*,#5644,.F.);
#7183=ORIENTED_EDGE('',*,*,#5631,.T.);
#7184=ORIENTED_EDGE('',*,*,#5586,.T.);
#7185=ORIENTED_EDGE('',*,*,#5645,.F.);
#7186=ORIENTED_EDGE('',*,*,#5646,.F.);
#7187=ORIENTED_EDGE('',*,*,#5643,.T.);
#7188=ORIENTED_EDGE('',*,*,#5585,.T.);
#7189=ORIENTED_EDGE('',*,*,#5647,.F.);
#7190=ORIENTED_EDGE('',*,*,#5648,.F.);
#7191=ORIENTED_EDGE('',*,*,#5645,.T.);
#7192=ORIENTED_EDGE('',*,*,#5584,.T.);
#7193=ORIENTED_EDGE('',*,*,#5598,.T.);
#7194=ORIENTED_EDGE('',*,*,#5649,.F.);
#7195=ORIENTED_EDGE('',*,*,#5567,.F.);
#7196=ORIENTED_EDGE('',*,*,#5650,.T.);
#7197=ORIENTED_EDGE('',*,*,#5651,.T.);
#7198=ORIENTED_EDGE('',*,*,#5652,.F.);
#7199=ORIENTED_EDGE('',*,*,#5647,.T.);
#7200=ORIENTED_EDGE('',*,*,#5652,.T.);
#7201=ORIENTED_EDGE('',*,*,#5653,.T.);
#7202=ORIENTED_EDGE('',*,*,#5637,.T.);
#7203=ORIENTED_EDGE('',*,*,#5642,.T.);
#7204=ORIENTED_EDGE('',*,*,#5632,.T.);
#7205=ORIENTED_EDGE('',*,*,#5644,.T.);
#7206=ORIENTED_EDGE('',*,*,#5646,.T.);
#7207=ORIENTED_EDGE('',*,*,#5648,.T.);
#7208=ORIENTED_EDGE('',*,*,#5597,.T.);
#7209=ORIENTED_EDGE('',*,*,#5640,.F.);
#7210=ORIENTED_EDGE('',*,*,#5560,.F.);
#7211=ORIENTED_EDGE('',*,*,#5654,.F.);
#7212=ORIENTED_EDGE('',*,*,#5655,.F.);
#7213=ORIENTED_EDGE('',*,*,#5656,.F.);
#7214=ORIENTED_EDGE('',*,*,#5657,.F.);
#7215=ORIENTED_EDGE('',*,*,#5658,.F.);
#7216=ORIENTED_EDGE('',*,*,#5568,.F.);
#7217=ORIENTED_EDGE('',*,*,#5649,.T.);
#7218=ORIENTED_EDGE('',*,*,#5556,.F.);
#7219=ORIENTED_EDGE('',*,*,#5653,.F.);
#7220=ORIENTED_EDGE('',*,*,#5651,.F.);
#7221=ORIENTED_EDGE('',*,*,#5659,.F.);
#7222=ORIENTED_EDGE('',*,*,#5638,.F.);
#7223=ORIENTED_EDGE('',*,*,#5659,.T.);
#7224=ORIENTED_EDGE('',*,*,#5650,.F.);
#7225=ORIENTED_EDGE('',*,*,#5566,.F.);
#7226=ORIENTED_EDGE('',*,*,#5660,.T.);
#7227=ORIENTED_EDGE('',*,*,#5661,.T.);
#7228=ORIENTED_EDGE('',*,*,#5662,.T.);
#7229=ORIENTED_EDGE('',*,*,#5663,.T.);
#7230=ORIENTED_EDGE('',*,*,#5664,.T.);
#7231=ORIENTED_EDGE('',*,*,#5562,.F.);
#7232=ORIENTED_EDGE('',*,*,#5639,.T.);
#7233=ORIENTED_EDGE('',*,*,#5665,.T.);
#7234=ORIENTED_EDGE('',*,*,#5666,.F.);
#7235=ORIENTED_EDGE('',*,*,#5660,.F.);
#7236=ORIENTED_EDGE('',*,*,#5565,.T.);
#7237=ORIENTED_EDGE('',*,*,#5667,.T.);
#7238=ORIENTED_EDGE('',*,*,#5668,.F.);
#7239=ORIENTED_EDGE('',*,*,#5661,.F.);
#7240=ORIENTED_EDGE('',*,*,#5666,.T.);
#7241=ORIENTED_EDGE('',*,*,#5669,.T.);
#7242=ORIENTED_EDGE('',*,*,#5670,.F.);
#7243=ORIENTED_EDGE('',*,*,#5662,.F.);
#7244=ORIENTED_EDGE('',*,*,#5668,.T.);
#7245=ORIENTED_EDGE('',*,*,#5671,.T.);
#7246=ORIENTED_EDGE('',*,*,#5672,.F.);
#7247=ORIENTED_EDGE('',*,*,#5663,.F.);
#7248=ORIENTED_EDGE('',*,*,#5670,.T.);
#7249=ORIENTED_EDGE('',*,*,#5673,.T.);
#7250=ORIENTED_EDGE('',*,*,#5563,.F.);
#7251=ORIENTED_EDGE('',*,*,#5664,.F.);
#7252=ORIENTED_EDGE('',*,*,#5672,.T.);
#7253=ORIENTED_EDGE('',*,*,#5665,.F.);
#7254=ORIENTED_EDGE('',*,*,#5564,.F.);
#7255=ORIENTED_EDGE('',*,*,#5673,.F.);
#7256=ORIENTED_EDGE('',*,*,#5671,.F.);
#7257=ORIENTED_EDGE('',*,*,#5669,.F.);
#7258=ORIENTED_EDGE('',*,*,#5667,.F.);
#7259=ORIENTED_EDGE('',*,*,#5550,.T.);
#7260=ORIENTED_EDGE('',*,*,#5553,.T.);
#7261=ORIENTED_EDGE('',*,*,#5658,.T.);
#7262=ORIENTED_EDGE('',*,*,#5674,.F.);
#7263=ORIENTED_EDGE('',*,*,#5675,.F.);
#7264=ORIENTED_EDGE('',*,*,#5557,.T.);
#7265=ORIENTED_EDGE('',*,*,#5657,.T.);
#7266=ORIENTED_EDGE('',*,*,#5676,.F.);
#7267=ORIENTED_EDGE('',*,*,#5677,.F.);
#7268=ORIENTED_EDGE('',*,*,#5674,.T.);
#7269=ORIENTED_EDGE('',*,*,#5656,.T.);
#7270=ORIENTED_EDGE('',*,*,#5678,.F.);
#7271=ORIENTED_EDGE('',*,*,#5679,.F.);
#7272=ORIENTED_EDGE('',*,*,#5676,.T.);
#7273=ORIENTED_EDGE('',*,*,#5655,.T.);
#7274=ORIENTED_EDGE('',*,*,#5680,.F.);
#7275=ORIENTED_EDGE('',*,*,#5681,.F.);
#7276=ORIENTED_EDGE('',*,*,#5678,.T.);
#7277=ORIENTED_EDGE('',*,*,#5654,.T.);
#7278=ORIENTED_EDGE('',*,*,#5559,.F.);
#7279=ORIENTED_EDGE('',*,*,#5682,.F.);
#7280=ORIENTED_EDGE('',*,*,#5680,.T.);
#7281=ORIENTED_EDGE('',*,*,#5675,.T.);
#7282=ORIENTED_EDGE('',*,*,#5677,.T.);
#7283=ORIENTED_EDGE('',*,*,#5679,.T.);
#7284=ORIENTED_EDGE('',*,*,#5681,.T.);
#7285=ORIENTED_EDGE('',*,*,#5682,.T.);
#7286=ORIENTED_EDGE('',*,*,#5558,.T.);
#7287=ORIENTED_EDGE('',*,*,#5554,.F.);
#7288=ORIENTED_EDGE('',*,*,#5577,.T.);
#7289=ORIENTED_EDGE('',*,*,#5610,.F.);
#7290=ORIENTED_EDGE('',*,*,#5630,.F.);
#7291=ORIENTED_EDGE('',*,*,#5683,.F.);
#7292=ORIENTED_EDGE('',*,*,#5624,.F.);
#7293=ORIENTED_EDGE('',*,*,#5684,.F.);
#7294=ORIENTED_EDGE('',*,*,#5616,.F.);
#7295=ORIENTED_EDGE('',*,*,#5604,.F.);
#7296=ORIENTED_EDGE('',*,*,#5601,.T.);
#7297=ORIENTED_EDGE('',*,*,#5613,.T.);
#7298=ORIENTED_EDGE('',*,*,#5685,.T.);
#7299=ORIENTED_EDGE('',*,*,#5620,.T.);
#7300=ORIENTED_EDGE('',*,*,#5686,.T.);
#7301=ORIENTED_EDGE('',*,*,#5627,.T.);
#7302=ORIENTED_EDGE('',*,*,#5607,.T.);
#7303=ORIENTED_EDGE('',*,*,#5571,.F.);
#7304=ORIENTED_EDGE('',*,*,#5687,.F.);
#7305=ORIENTED_EDGE('',*,*,#5617,.T.);
#7306=ORIENTED_EDGE('',*,*,#5685,.F.);
#7307=ORIENTED_EDGE('',*,*,#5612,.F.);
#7308=ORIENTED_EDGE('',*,*,#5688,.F.);
#7309=ORIENTED_EDGE('',*,*,#5580,.T.);
#7310=ORIENTED_EDGE('',*,*,#5689,.T.);
#7311=ORIENTED_EDGE('',*,*,#5614,.F.);
#7312=ORIENTED_EDGE('',*,*,#5684,.T.);
#7313=ORIENTED_EDGE('',*,*,#5623,.T.);
#7314=ORIENTED_EDGE('',*,*,#5690,.T.);
#7315=ORIENTED_EDGE('',*,*,#5691,.F.);
#7316=ORIENTED_EDGE('',*,*,#5592,.F.);
#7317=ORIENTED_EDGE('',*,*,#5595,.F.);
#7318=ORIENTED_EDGE('',*,*,#5692,.T.);
#7319=ORIENTED_EDGE('',*,*,#5625,.T.);
#7320=ORIENTED_EDGE('',*,*,#5686,.F.);
#7321=ORIENTED_EDGE('',*,*,#5619,.F.);
#7322=ORIENTED_EDGE('',*,*,#5693,.T.);
#7323=ORIENTED_EDGE('',*,*,#5593,.F.);
#7324=ORIENTED_EDGE('',*,*,#5582,.F.);
#7325=ORIENTED_EDGE('',*,*,#5694,.F.);
#7326=ORIENTED_EDGE('',*,*,#5695,.F.);
#7327=ORIENTED_EDGE('',*,*,#5621,.F.);
#7328=ORIENTED_EDGE('',*,*,#5683,.T.);
#7329=ORIENTED_EDGE('',*,*,#5629,.T.);
#7330=ORIENTED_EDGE('',*,*,#5696,.F.);
#7331=ORIENTED_EDGE('',*,*,#5574,.T.);
#7332=ORIENTED_EDGE('',*,*,#5551,.F.);
#7333=ORIENTED_EDGE('',*,*,#5548,.F.);
#7334=ORIENTED_EDGE('',*,*,#5634,.T.);
#7335=ORIENTED_EDGE('',*,*,#5545,.T.);
#7336=ORIENTED_EDGE('',*,*,#5547,.T.);
#7337=ORIENTED_EDGE('',*,*,#5636,.T.);
#7338=ORIENTED_EDGE('',*,*,#5540,.T.);
#7339=ORIENTED_EDGE('',*,*,#5542,.T.);
#7340=ORIENTED_EDGE('',*,*,#5635,.T.);
#7341=ORIENTED_EDGE('',*,*,#5535,.T.);
#7342=ORIENTED_EDGE('',*,*,#5537,.T.);
#7343=ORIENTED_EDGE('',*,*,#5573,.T.);
#7344=ORIENTED_EDGE('',*,*,#5606,.F.);
#7345=ORIENTED_EDGE('',*,*,#5626,.F.);
#7346=ORIENTED_EDGE('',*,*,#5692,.F.);
#7347=ORIENTED_EDGE('',*,*,#5575,.T.);
#7348=ORIENTED_EDGE('',*,*,#5696,.T.);
#7349=ORIENTED_EDGE('',*,*,#5628,.F.);
#7350=ORIENTED_EDGE('',*,*,#5608,.F.);
#7351=ORIENTED_EDGE('',*,*,#5695,.T.);
#7352=ORIENTED_EDGE('',*,*,#5697,.F.);
#7353=ORIENTED_EDGE('',*,*,#5690,.F.);
#7354=ORIENTED_EDGE('',*,*,#5622,.F.);
#7355=ORIENTED_EDGE('',*,*,#5693,.F.);
#7356=ORIENTED_EDGE('',*,*,#5618,.F.);
#7357=ORIENTED_EDGE('',*,*,#5687,.T.);
#7358=ORIENTED_EDGE('',*,*,#5594,.F.);
#7359=ORIENTED_EDGE('',*,*,#5691,.T.);
#7360=ORIENTED_EDGE('',*,*,#5697,.T.);
#7361=ORIENTED_EDGE('',*,*,#5694,.T.);
#7362=ORIENTED_EDGE('',*,*,#5581,.F.);
#7363=ORIENTED_EDGE('',*,*,#5569,.T.);
#7364=ORIENTED_EDGE('',*,*,#5688,.T.);
#7365=ORIENTED_EDGE('',*,*,#5611,.F.);
#7366=ORIENTED_EDGE('',*,*,#5599,.F.);
#7367=ORIENTED_EDGE('',*,*,#5579,.T.);
#7368=ORIENTED_EDGE('',*,*,#5603,.F.);
#7369=ORIENTED_EDGE('',*,*,#5615,.F.);
#7370=ORIENTED_EDGE('',*,*,#5689,.F.);
#9178=CYLINDRICAL_SURFACE('',#10190,2.59999999999999);
#9179=CYLINDRICAL_SURFACE('',#10195,2.59999999999999);
#9180=CYLINDRICAL_SURFACE('',#10200,2.59999999999999);
#9181=CYLINDRICAL_SURFACE('',#10205,2.5);
#9182=CYLINDRICAL_SURFACE('',#10208,2.5);
#9183=CYLINDRICAL_SURFACE('',#10211,9.1);
#9322=ADVANCED_FACE('',(#997),#9178,.F.);
#9323=ADVANCED_FACE('',(#998),#9179,.F.);
#9324=ADVANCED_FACE('',(#999),#9180,.F.);
#9325=ADVANCED_FACE('',(#1000),#9181,.F.);
#9326=ADVANCED_FACE('',(#1001),#9182,.F.);
#9327=ADVANCED_FACE('',(#1002),#9183,.F.);
#9328=ADVANCED_FACE('',(#1003,#320),#506,.F.);
#9329=ADVANCED_FACE('',(#1004),#507,.T.);
#9330=ADVANCED_FACE('',(#1005),#508,.T.);
#9331=ADVANCED_FACE('',(#1006),#509,.T.);
#9332=ADVANCED_FACE('',(#1007),#510,.T.);
#9333=ADVANCED_FACE('',(#1008),#511,.T.);
#9334=ADVANCED_FACE('',(#1009),#512,.T.);
#9335=ADVANCED_FACE('',(#1010),#513,.T.);
#9336=ADVANCED_FACE('',(#1011),#514,.T.);
#9337=ADVANCED_FACE('',(#1012),#515,.T.);
#9338=ADVANCED_FACE('',(#1013),#516,.T.);
#9339=ADVANCED_FACE('',(#1014),#517,.T.);
#9340=ADVANCED_FACE('',(#1015),#518,.T.);
#9341=ADVANCED_FACE('',(#1016,#321,#322,#323),#519,.F.);
#9342=ADVANCED_FACE('',(#1017,#324,#325,#326),#520,.F.);
#9343=ADVANCED_FACE('',(#1018),#521,.F.);
#9344=ADVANCED_FACE('',(#1019),#522,.F.);
#9345=ADVANCED_FACE('',(#1020),#523,.F.);
#9346=ADVANCED_FACE('',(#1021),#524,.F.);
#9347=ADVANCED_FACE('',(#1022),#525,.F.);
#9348=ADVANCED_FACE('',(#1023),#526,.F.);
#9349=ADVANCED_FACE('',(#1024,#327),#527,.F.);
#9350=ADVANCED_FACE('',(#1025),#528,.T.);
#9351=ADVANCED_FACE('',(#1026),#529,.F.);
#9352=ADVANCED_FACE('',(#1027),#530,.F.);
#9353=ADVANCED_FACE('',(#1028),#531,.F.);
#9354=ADVANCED_FACE('',(#1029),#532,.F.);
#9355=ADVANCED_FACE('',(#1030),#533,.F.);
#9356=ADVANCED_FACE('',(#1031),#534,.F.);
#9357=ADVANCED_FACE('',(#1032,#328,#329),#535,.T.);
#9358=ADVANCED_FACE('',(#1033),#536,.F.);
#9359=ADVANCED_FACE('',(#1034),#537,.F.);
#9360=ADVANCED_FACE('',(#1035),#538,.F.);
#9361=ADVANCED_FACE('',(#1036),#539,.F.);
#9362=ADVANCED_FACE('',(#1037),#540,.F.);
#9363=ADVANCED_FACE('',(#1038,#330),#541,.F.);
#9364=ADVANCED_FACE('',(#1039),#542,.T.);
#9365=ADVANCED_FACE('',(#1040),#543,.F.);
#9366=ADVANCED_FACE('',(#1041),#544,.T.);
#9367=ADVANCED_FACE('',(#1042),#545,.T.);
#9368=ADVANCED_FACE('',(#1043),#546,.F.);
#9369=ADVANCED_FACE('',(#1044),#547,.F.);
#9370=ADVANCED_FACE('',(#1045),#548,.T.);
#9371=ADVANCED_FACE('',(#1046),#549,.T.);
#9372=ADVANCED_FACE('',(#1047),#550,.T.);
#9373=ADVANCED_FACE('',(#1048),#551,.T.);
#9374=ADVANCED_FACE('',(#1049),#552,.T.);
#9375=ADVANCED_FACE('',(#1050),#553,.T.);
#9376=ADVANCED_FACE('',(#1051),#554,.T.);
#9377=ADVANCED_FACE('',(#1052),#555,.T.);
#9378=ADVANCED_FACE('',(#1053),#556,.T.);
#9379=ADVANCED_FACE('',(#1054),#557,.T.);
#9789=CLOSED_SHELL('',(#9322,#9323,#9324,#9325,#9326,#9327,#9328,#9329,
#9330,#9331,#9332,#9333,#9334,#9335,#9336,#9337,#9338,#9339,#9340,#9341,
#9342,#9343,#9344,#9345,#9346,#9347,#9348,#9349,#9350,#9351,#9352,#9353,
#9354,#9355,#9356,#9357,#9358,#9359,#9360,#9361,#9362,#9363,#9364,#9365,
#9366,#9367,#9368,#9369,#9370,#9371,#9372,#9373,#9374,#9375,#9376,#9377,
#9378,#9379));
#10189=AXIS2_PLACEMENT_3D('',#14139,#11352,#11353);
#10190=AXIS2_PLACEMENT_3D('',#14140,#11354,#11355);
#10191=AXIS2_PLACEMENT_3D('',#14142,#11356,#11357);
#10192=AXIS2_PLACEMENT_3D('',#14146,#11359,#11360);
#10193=AXIS2_PLACEMENT_3D('',#14148,#11361,#11362);
#10194=AXIS2_PLACEMENT_3D('',#14149,#11363,#11364);
#10195=AXIS2_PLACEMENT_3D('',#14150,#11365,#11366);
#10196=AXIS2_PLACEMENT_3D('',#14152,#11367,#11368);
#10197=AXIS2_PLACEMENT_3D('',#14156,#11370,#11371);
#10198=AXIS2_PLACEMENT_3D('',#14158,#11372,#11373);
#10199=AXIS2_PLACEMENT_3D('',#14159,#11374,#11375);
#10200=AXIS2_PLACEMENT_3D('',#14160,#11376,#11377);
#10201=AXIS2_PLACEMENT_3D('',#14162,#11378,#11379);
#10202=AXIS2_PLACEMENT_3D('',#14166,#11381,#11382);
#10203=AXIS2_PLACEMENT_3D('',#14168,#11383,#11384);
#10204=AXIS2_PLACEMENT_3D('',#14169,#11385,#11386);
#10205=AXIS2_PLACEMENT_3D('',#14170,#11387,#11388);
#10206=AXIS2_PLACEMENT_3D('',#14172,#11389,#11390);
#10207=AXIS2_PLACEMENT_3D('',#14175,#11392,#11393);
#10208=AXIS2_PLACEMENT_3D('',#14176,#11394,#11395);
#10209=AXIS2_PLACEMENT_3D('',#14178,#11396,#11397);
#10210=AXIS2_PLACEMENT_3D('',#14181,#11399,#11400);
#10211=AXIS2_PLACEMENT_3D('',#14182,#11401,#11402);
#10212=AXIS2_PLACEMENT_3D('',#14184,#11403,#11404);
#10213=AXIS2_PLACEMENT_3D('',#14187,#11406,#11407);
#10214=AXIS2_PLACEMENT_3D('',#14188,#11408,#11409);
#10215=AXIS2_PLACEMENT_3D('',#14237,#11434,#11435);
#10216=AXIS2_PLACEMENT_3D('',#14262,#11448,#11449);
#10217=AXIS2_PLACEMENT_3D('',#14273,#11456,#11457);
#10218=AXIS2_PLACEMENT_3D('',#14279,#11461,#11462);
#10219=AXIS2_PLACEMENT_3D('',#14285,#11466,#11467);
#10220=AXIS2_PLACEMENT_3D('',#14291,#11471,#11472);
#10221=AXIS2_PLACEMENT_3D('',#14297,#11476,#11477);
#10222=AXIS2_PLACEMENT_3D('',#14303,#11481,#11482);
#10223=AXIS2_PLACEMENT_3D('',#14309,#11486,#11487);
#10224=AXIS2_PLACEMENT_3D('',#14318,#11492,#11493);
#10225=AXIS2_PLACEMENT_3D('',#14327,#11498,#11499);
#10226=AXIS2_PLACEMENT_3D('',#14333,#11503,#11504);
#10227=AXIS2_PLACEMENT_3D('',#14339,#11508,#11509);
#10228=AXIS2_PLACEMENT_3D('',#14348,#11516,#11517);
#10229=AXIS2_PLACEMENT_3D('',#14357,#11523,#11524);
#10230=AXIS2_PLACEMENT_3D('',#14359,#11526,#11527);
#10231=AXIS2_PLACEMENT_3D('',#14363,#11530,#11531);
#10232=AXIS2_PLACEMENT_3D('',#14367,#11534,#11535);
#10233=AXIS2_PLACEMENT_3D('',#14371,#11538,#11539);
#10234=AXIS2_PLACEMENT_3D('',#14378,#11544,#11545);
#10235=AXIS2_PLACEMENT_3D('',#14380,#11547,#11548);
#10236=AXIS2_PLACEMENT_3D('',#14390,#11554,#11555);
#10237=AXIS2_PLACEMENT_3D('',#14392,#11557,#11558);
#10238=AXIS2_PLACEMENT_3D('',#14402,#11564,#11565);
#10239=AXIS2_PLACEMENT_3D('',#14406,#11568,#11569);
#10240=AXIS2_PLACEMENT_3D('',#14410,#11572,#11573);
#10241=AXIS2_PLACEMENT_3D('',#14414,#11576,#11577);
#10242=AXIS2_PLACEMENT_3D('',#14418,#11580,#11581);
#10243=AXIS2_PLACEMENT_3D('',#14420,#11583,#11584);
#10244=AXIS2_PLACEMENT_3D('',#14421,#11585,#11586);
#10245=AXIS2_PLACEMENT_3D('',#14425,#11589,#11590);
#10246=AXIS2_PLACEMENT_3D('',#14429,#11593,#11594);
#10247=AXIS2_PLACEMENT_3D('',#14433,#11597,#11598);
#10248=AXIS2_PLACEMENT_3D('',#14437,#11601,#11602);
#10249=AXIS2_PLACEMENT_3D('',#14439,#11604,#11605);
#10250=AXIS2_PLACEMENT_3D('',#14440,#11606,#11607);
#10251=AXIS2_PLACEMENT_3D('',#14443,#11610,#11611);
#10252=AXIS2_PLACEMENT_3D('',#14446,#11614,#11615);
#10253=AXIS2_PLACEMENT_3D('',#14453,#11621,#11622);
#10254=AXIS2_PLACEMENT_3D('',#14460,#11628,#11629);
#10255=AXIS2_PLACEMENT_3D('',#14461,#11630,#11631);
#10256=AXIS2_PLACEMENT_3D('',#14462,#11632,#11633);
#10257=AXIS2_PLACEMENT_3D('',#14463,#11634,#11635);
#10258=AXIS2_PLACEMENT_3D('',#14464,#11636,#11637);
#10259=AXIS2_PLACEMENT_3D('',#14465,#11638,#11639);
#10260=AXIS2_PLACEMENT_3D('',#14466,#11640,#11641);
#10261=AXIS2_PLACEMENT_3D('',#14467,#11642,#11643);
#10262=AXIS2_PLACEMENT_3D('',#14469,#11645,#11646);
#10263=AXIS2_PLACEMENT_3D('',#14470,#11647,#11648);
#10264=AXIS2_PLACEMENT_3D('',#14471,#11649,#11650);
#10265=AXIS2_PLACEMENT_3D('',#14472,#11651,#11652);
#11352=DIRECTION('axis',(0.,0.,1.));
#11353=DIRECTION('refdir',(1.,0.,0.));
#11354=DIRECTION('center_axis',(-1.,0.,0.));
#11355=DIRECTION('ref_axis',(0.,0.,1.));
#11356=DIRECTION('center_axis',(1.,0.,0.));
#11357=DIRECTION('ref_axis',(0.,0.,1.));
#11358=DIRECTION('',(-1.,0.,0.));
#11359=DIRECTION('center_axis',(1.,0.,0.));
#11360=DIRECTION('ref_axis',(0.,0.,-1.));
#11361=DIRECTION('center_axis',(-0.832050294337839,-8.41209314899718E-15,
0.554700196225236));
#11362=DIRECTION('ref_axis',(0.554700196225236,1.57539479552213E-13,0.832050294337839));
#11363=DIRECTION('center_axis',(1.,0.,0.));
#11364=DIRECTION('ref_axis',(0.,0.,-1.));
#11365=DIRECTION('center_axis',(-1.,0.,0.));
#11366=DIRECTION('ref_axis',(0.,0.,1.));
#11367=DIRECTION('center_axis',(1.,0.,0.));
#11368=DIRECTION('ref_axis',(0.,0.,1.));
#11369=DIRECTION('',(-1.,0.,0.));
#11370=DIRECTION('center_axis',(1.,0.,0.));
#11371=DIRECTION('ref_axis',(0.,0.,-1.));
#11372=DIRECTION('center_axis',(-0.832050294337839,-8.56787265175636E-15,
0.554700196225237));
#11373=DIRECTION('ref_axis',(0.554700196225236,7.46312953944725E-13,0.832050294337839));
#11374=DIRECTION('center_axis',(1.,0.,0.));
#11375=DIRECTION('ref_axis',(0.,0.,-1.));
#11376=DIRECTION('center_axis',(-1.,0.,0.));
#11377=DIRECTION('ref_axis',(0.,0.,1.));
#11378=DIRECTION('center_axis',(1.,0.,0.));
#11379=DIRECTION('ref_axis',(0.,0.,1.));
#11380=DIRECTION('',(-1.,0.,0.));
#11381=DIRECTION('center_axis',(1.,0.,0.));
#11382=DIRECTION('ref_axis',(0.,0.,-1.));
#11383=DIRECTION('center_axis',(-0.832050294337839,-8.56787265175632E-15,
0.554700196225236));
#11384=DIRECTION('ref_axis',(0.554700196225236,4.28606070402036E-13,0.832050294337839));
#11385=DIRECTION('center_axis',(1.,0.,0.));
#11386=DIRECTION('ref_axis',(0.,0.,-1.));
#11387=DIRECTION('center_axis',(0.,-1.,0.));
#11388=DIRECTION('ref_axis',(0.,0.,-1.));
#11389=DIRECTION('center_axis',(0.,1.,0.));
#11390=DIRECTION('ref_axis',(0.,0.,1.));
#11391=DIRECTION('',(0.,-1.,0.));
#11392=DIRECTION('center_axis',(0.,1.,0.));
#11393=DIRECTION('ref_axis',(0.,0.,-1.));
#11394=DIRECTION('center_axis',(0.,-1.,0.));
#11395=DIRECTION('ref_axis',(0.,0.,-1.));
#11396=DIRECTION('center_axis',(0.,1.,0.));
#11397=DIRECTION('ref_axis',(0.,0.,1.));
#11398=DIRECTION('',(0.,-1.,0.));
#11399=DIRECTION('center_axis',(0.,1.,0.));
#11400=DIRECTION('ref_axis',(0.,0.,-1.));
#11401=DIRECTION('center_axis',(0.,-1.,0.));
#11402=DIRECTION('ref_axis',(0.,0.,-1.));
#11403=DIRECTION('center_axis',(0.,1.,0.));
#11404=DIRECTION('ref_axis',(0.,0.,-1.));
#11405=DIRECTION('',(0.,-1.,0.));
#11406=DIRECTION('center_axis',(0.,-1.,0.));
#11407=DIRECTION('ref_axis',(0.,0.,1.));
#11408=DIRECTION('center_axis',(0.,0.,-1.));
#11409=DIRECTION('ref_axis',(-1.,0.,0.));
#11410=DIRECTION('',(0.,-1.,0.));
#11411=DIRECTION('',(-1.,0.,0.));
#11412=DIRECTION('',(0.,-1.,0.));
#11413=DIRECTION('',(1.,0.,0.));
#11414=DIRECTION('',(0.,-1.,0.));
#11415=DIRECTION('',(-1.,0.,0.));
#11416=DIRECTION('',(0.,-1.,0.));
#11417=DIRECTION('',(-1.,0.,0.));
#11418=DIRECTION('',(0.,-1.,0.));
#11419=DIRECTION('',(-1.,0.,0.));
#11420=DIRECTION('',(0.,-1.,0.));
#11421=DIRECTION('',(1.,0.,0.));
#11422=DIRECTION('',(1.,0.,0.));
#11423=DIRECTION('',(0.,1.,0.));
#11424=DIRECTION('',(-1.,0.,0.));
#11425=DIRECTION('',(0.,-1.,0.));
#11426=DIRECTION('',(1.,0.,0.));
#11427=DIRECTION('',(0.,-1.,0.));
#11428=DIRECTION('',(-1.,0.,0.));
#11429=DIRECTION('',(0.,-1.,0.));
#11430=DIRECTION('',(-1.,0.,0.));
#11431=DIRECTION('',(0.,1.,0.));
#11432=DIRECTION('',(-1.,0.,0.));
#11433=DIRECTION('',(0.,1.,0.));
#11434=DIRECTION('center_axis',(0.,-1.,0.));
#11435=DIRECTION('ref_axis',(0.,0.,-1.));
#11436=DIRECTION('',(-1.,0.,0.));
#11437=DIRECTION('',(0.,0.,1.));
#11438=DIRECTION('',(1.,0.,0.));
#11439=DIRECTION('',(0.,0.,1.));
#11440=DIRECTION('',(-1.,0.,0.));
#11441=DIRECTION('',(0.554700196225229,0.,-0.832050294337844));
#11442=DIRECTION('',(-1.,0.,0.));
#11443=DIRECTION('',(0.554700196225229,0.,0.832050294337844));
#11444=DIRECTION('',(-1.,0.,0.));
#11445=DIRECTION('',(0.,0.,-1.));
#11446=DIRECTION('',(1.,0.,0.));
#11447=DIRECTION('',(0.,0.,-1.));
#11448=DIRECTION('center_axis',(0.,0.,-1.));
#11449=DIRECTION('ref_axis',(-1.,0.,0.));
#11450=DIRECTION('',(0.,-1.,0.));
#11451=DIRECTION('',(1.,0.,0.));
#11452=DIRECTION('',(0.,1.,0.));
#11453=DIRECTION('',(0.,1.,0.));
#11454=DIRECTION('',(1.,0.,0.));
#11455=DIRECTION('',(0.,-1.,0.));
#11456=DIRECTION('center_axis',(-1.,0.,0.));
#11457=DIRECTION('ref_axis',(0.,0.,1.));
#11458=DIRECTION('',(0.,0.,-1.));
#11459=DIRECTION('',(0.,-1.,0.));
#11460=DIRECTION('',(0.,0.,-1.));
#11461=DIRECTION('center_axis',(-1.,0.,0.));
#11462=DIRECTION('ref_axis',(0.,0.,1.));
#11463=DIRECTION('',(0.,-1.,0.));
#11464=DIRECTION('',(0.,0.,1.));
#11465=DIRECTION('',(0.,0.,-1.));
#11466=DIRECTION('center_axis',(1.,0.,0.));
#11467=DIRECTION('ref_axis',(0.,0.,-1.));
#11468=DIRECTION('',(0.,-1.,0.));
#11469=DIRECTION('',(0.,0.,1.));
#11470=DIRECTION('',(0.,0.,1.));
#11471=DIRECTION('center_axis',(1.,0.,0.));
#11472=DIRECTION('ref_axis',(0.,0.,-1.));
#11473=DIRECTION('',(0.,0.,-1.));
#11474=DIRECTION('',(0.,-1.,0.));
#11475=DIRECTION('',(0.,0.,1.));
#11476=DIRECTION('center_axis',(0.,0.,-1.));
#11477=DIRECTION('ref_axis',(-1.,0.,0.));
#11478=DIRECTION('',(1.,0.,0.));
#11479=DIRECTION('',(0.,-1.,0.));
#11480=DIRECTION('',(1.,0.,0.));
#11481=DIRECTION('center_axis',(0.,0.,-1.));
#11482=DIRECTION('ref_axis',(-1.,0.,0.));
#11483=DIRECTION('',(0.,-1.,0.));
#11484=DIRECTION('',(-1.,0.,0.));
#11485=DIRECTION('',(1.,0.,0.));
#11486=DIRECTION('center_axis',(0.,0.,1.));
#11487=DIRECTION('ref_axis',(1.,0.,0.));
#11488=DIRECTION('',(0.,-1.,0.));
#11489=DIRECTION('',(-1.,0.,0.));
#11490=DIRECTION('',(0.,-1.,0.));
#11491=DIRECTION('',(-1.,0.,0.));
#11492=DIRECTION('center_axis',(0.,0.,1.));
#11493=DIRECTION('ref_axis',(1.,0.,0.));
#11494=DIRECTION('',(0.,-1.,0.));
#11495=DIRECTION('',(1.,0.,0.));
#11496=DIRECTION('',(0.,-1.,0.));
#11497=DIRECTION('',(-1.,0.,0.));
#11498=DIRECTION('center_axis',(0.,0.,-1.));
#11499=DIRECTION('ref_axis',(-1.,0.,0.));
#11500=DIRECTION('',(0.,-1.,0.));
#11501=DIRECTION('',(1.,0.,0.));
#11502=DIRECTION('',(1.,0.,0.));
#11503=DIRECTION('center_axis',(0.,0.,-1.));
#11504=DIRECTION('ref_axis',(-1.,0.,0.));
#11505=DIRECTION('',(-1.,0.,0.));
#11506=DIRECTION('',(0.,-1.,0.));
#11507=DIRECTION('',(1.,0.,0.));
#11508=DIRECTION('center_axis',(0.832050294337844,0.,-0.554700196225229));
#11509=DIRECTION('ref_axis',(-0.554700196225229,0.,-0.832050294337844));
#11510=DIRECTION('',(0.,-1.,0.));
#11511=DIRECTION('',(0.554700196225229,0.,0.832050294337844));
#11512=DIRECTION('',(0.,-1.,0.));
#11513=DIRECTION('',(0.,-1.,0.));
#11514=DIRECTION('',(0.,-1.,0.));
#11515=DIRECTION('',(0.,-1.,0.));
#11516=DIRECTION('center_axis',(-1.,0.,0.));
#11517=DIRECTION('ref_axis',(0.,0.,1.));
#11518=DIRECTION('',(0.,0.,-1.));
#11519=DIRECTION('',(0.,1.,0.));
#11520=DIRECTION('',(0.,0.,-1.));
#11521=DIRECTION('',(0.,0.,-1.));
#11522=DIRECTION('',(0.,-1.,0.));
#11523=DIRECTION('center_axis',(0.,0.,1.));
#11524=DIRECTION('ref_axis',(1.,0.,0.));
#11525=DIRECTION('',(-1.,0.,0.));
#11526=DIRECTION('center_axis',(0.,0.,1.));
#11527=DIRECTION('ref_axis',(1.,0.,0.));
#11528=DIRECTION('',(0.,-1.,0.));
#11529=DIRECTION('',(-1.,0.,0.));
#11530=DIRECTION('center_axis',(-0.832050294337844,0.,-0.554700196225229));
#11531=DIRECTION('ref_axis',(-0.554700196225229,0.,0.832050294337844));
#11532=DIRECTION('',(0.,-1.,0.));
#11533=DIRECTION('',(0.554700196225229,0.,-0.832050294337844));
#11534=DIRECTION('center_axis',(0.,0.,1.));
#11535=DIRECTION('ref_axis',(1.,0.,0.));
#11536=DIRECTION('',(0.,-1.,0.));
#11537=DIRECTION('',(-1.,0.,0.));
#11538=DIRECTION('center_axis',(1.,0.,0.));
#11539=DIRECTION('ref_axis',(0.,0.,-1.));
#11540=DIRECTION('',(0.,0.,-1.));
#11541=DIRECTION('',(0.,0.,-1.));
#11542=DIRECTION('',(0.,-1.,0.));
#11543=DIRECTION('',(0.,0.,1.));
#11544=DIRECTION('center_axis',(0.,-1.,0.));
#11545=DIRECTION('ref_axis',(0.,0.,-1.));
#11546=DIRECTION('',(1.,0.,0.));
#11547=DIRECTION('center_axis',(0.,1.,0.));
#11548=DIRECTION('ref_axis',(0.,0.,1.));
#11549=DIRECTION('',(0.,0.,-1.));
#11550=DIRECTION('',(0.70710678118653,0.,-0.707106781186565));
#11551=DIRECTION('',(1.,0.,0.));
#11552=DIRECTION('',(0.707106781186556,0.,0.707106781186539));
#11553=DIRECTION('',(0.,0.,1.));
#11554=DIRECTION('center_axis',(0.,0.,-1.));
#11555=DIRECTION('ref_axis',(-1.,0.,0.));
#11556=DIRECTION('',(-1.,0.,0.));
#11557=DIRECTION('center_axis',(0.,-1.,0.));
#11558=DIRECTION('ref_axis',(0.,0.,-1.));
#11559=DIRECTION('',(0.,0.,1.));
#11560=DIRECTION('',(0.707106781186555,0.,0.70710678118654));
#11561=DIRECTION('',(1.,0.,0.));
#11562=DIRECTION('',(0.70710678118653,0.,-0.707106781186565));
#11563=DIRECTION('',(0.,0.,-1.));
#11564=DIRECTION('center_axis',(1.,0.,0.));
#11565=DIRECTION('ref_axis',(0.,0.,-1.));
#11566=DIRECTION('',(0.,0.,1.));
#11567=DIRECTION('',(0.,-1.,0.));
#11568=DIRECTION('center_axis',(0.70710678118654,0.,-0.707106781186555));
#11569=DIRECTION('ref_axis',(-0.707106781186555,0.,-0.70710678118654));
#11570=DIRECTION('',(0.707106781186555,0.,0.70710678118654));
#11571=DIRECTION('',(0.,-1.,0.));
#11572=DIRECTION('center_axis',(0.,0.,-1.));
#11573=DIRECTION('ref_axis',(-1.,0.,0.));
#11574=DIRECTION('',(1.,0.,0.));
#11575=DIRECTION('',(0.,-1.,0.));
#11576=DIRECTION('center_axis',(-0.707106781186565,0.,-0.70710678118653));
#11577=DIRECTION('ref_axis',(-0.70710678118653,0.,0.707106781186565));
#11578=DIRECTION('',(0.70710678118653,0.,-0.707106781186565));
#11579=DIRECTION('',(0.,-1.,0.));
#11580=DIRECTION('center_axis',(-1.,0.,0.));
#11581=DIRECTION('ref_axis',(0.,0.,1.));
#11582=DIRECTION('',(0.,0.,-1.));
#11583=DIRECTION('center_axis',(0.,-1.,0.));
#11584=DIRECTION('ref_axis',(0.,0.,-1.));
#11585=DIRECTION('center_axis',(1.,0.,0.));
#11586=DIRECTION('ref_axis',(0.,0.,-1.));
#11587=DIRECTION('',(0.,-1.,0.));
#11588=DIRECTION('',(0.,0.,1.));
#11589=DIRECTION('center_axis',(0.707106781186539,0.,-0.707106781186556));
#11590=DIRECTION('ref_axis',(-0.707106781186556,0.,-0.707106781186539));
#11591=DIRECTION('',(0.,-1.,0.));
#11592=DIRECTION('',(0.707106781186556,0.,0.707106781186539));
#11593=DIRECTION('center_axis',(0.,0.,-1.));
#11594=DIRECTION('ref_axis',(-1.,0.,0.));
#11595=DIRECTION('',(0.,-1.,0.));
#11596=DIRECTION('',(1.,0.,0.));
#11597=DIRECTION('center_axis',(-0.707106781186565,0.,-0.70710678118653));
#11598=DIRECTION('ref_axis',(-0.70710678118653,0.,0.707106781186565));
#11599=DIRECTION('',(0.,-1.,0.));
#11600=DIRECTION('',(0.70710678118653,0.,-0.707106781186565));
#11601=DIRECTION('center_axis',(-1.,0.,0.));
#11602=DIRECTION('ref_axis',(0.,0.,1.));
#11603=DIRECTION('',(0.,0.,-1.));
#11604=DIRECTION('center_axis',(0.,-1.,0.));
#11605=DIRECTION('ref_axis',(0.,0.,-1.));
#11606=DIRECTION('center_axis',(0.,-1.,0.));
#11607=DIRECTION('ref_axis',(0.,0.,-1.));
#11608=DIRECTION('',(0.,0.,1.));
#11609=DIRECTION('',(0.,0.,-1.));
#11610=DIRECTION('center_axis',(0.,-1.,0.));
#11611=DIRECTION('ref_axis',(0.,0.,-1.));
#11612=DIRECTION('',(0.,0.,-1.));
#11613=DIRECTION('',(0.,0.,1.));
#11614=DIRECTION('center_axis',(-1.,0.,0.));
#11615=DIRECTION('ref_axis',(0.,0.,1.));
#11616=DIRECTION('',(0.,0.,-1.));
#11617=DIRECTION('',(0.,0.,-1.));
#11618=DIRECTION('',(0.,0.,-1.));
#11619=DIRECTION('',(0.,0.,-1.));
#11620=DIRECTION('',(0.,1.,0.));
#11621=DIRECTION('center_axis',(1.,0.,0.));
#11622=DIRECTION('ref_axis',(0.,0.,-1.));
#11623=DIRECTION('',(0.,0.,-1.));
#11624=DIRECTION('',(0.,0.,-1.));
#11625=DIRECTION('',(0.,-1.,0.));
#11626=DIRECTION('',(0.,0.,-1.));
#11627=DIRECTION('',(0.,0.,-1.));
#11628=DIRECTION('center_axis',(0.,1.,0.));
#11629=DIRECTION('ref_axis',(0.,0.,1.));
#11630=DIRECTION('center_axis',(0.,1.,0.));
#11631=DIRECTION('ref_axis',(0.,0.,1.));
#11632=DIRECTION('center_axis',(1.,0.,0.));
#11633=DIRECTION('ref_axis',(0.,0.,-1.));
#11634=DIRECTION('center_axis',(1.,0.,0.));
#11635=DIRECTION('ref_axis',(0.,0.,-1.));
#11636=DIRECTION('center_axis',(1.,0.,0.));
#11637=DIRECTION('ref_axis',(0.,0.,-1.));
#11638=DIRECTION('center_axis',(0.,1.,0.));
#11639=DIRECTION('ref_axis',(0.,0.,1.));
#11640=DIRECTION('center_axis',(0.,-1.,0.));
#11641=DIRECTION('ref_axis',(0.,0.,-1.));
#11642=DIRECTION('center_axis',(0.,-1.,0.));
#11643=DIRECTION('ref_axis',(0.,0.,-1.));
#11644=DIRECTION('',(-1.,0.,0.));
#11645=DIRECTION('center_axis',(0.,1.,0.));
#11646=DIRECTION('ref_axis',(0.,0.,1.));
#11647=DIRECTION('center_axis',(0.,0.,1.));
#11648=DIRECTION('ref_axis',(1.,0.,0.));
#11649=DIRECTION('center_axis',(0.,1.,0.));
#11650=DIRECTION('ref_axis',(0.,0.,1.));
#11651=DIRECTION('center_axis',(0.,-1.,0.));
#11652=DIRECTION('ref_axis',(0.,0.,-1.));
#14139=CARTESIAN_POINT('',(0.,0.,0.));
#14140=CARTESIAN_POINT('Origin',(58.,-36.,60.));
#14141=CARTESIAN_POINT('',(56.,-36.,57.4));
#14142=CARTESIAN_POINT('Origin',(56.,-36.,60.));
#14143=CARTESIAN_POINT('',(43.,-36.,57.4));
#14144=CARTESIAN_POINT('',(58.,-36.,57.4));
#14145=CARTESIAN_POINT('',(43.,-38.5941038915202,59.825));
#14146=CARTESIAN_POINT('Origin',(43.,-36.,60.));
#14147=CARTESIAN_POINT('',(43.,-33.4058961084799,59.825));
#14148=CARTESIAN_POINT('Origin',(43.1166666666667,-36.0000000000003,60.0000000000001));
#14149=CARTESIAN_POINT('Origin',(43.,-36.,60.));
#14150=CARTESIAN_POINT('Origin',(58.,0.,60.));
#14151=CARTESIAN_POINT('',(56.,-3.18408167778311E-16,57.4));
#14152=CARTESIAN_POINT('Origin',(56.,0.,60.));
#14153=CARTESIAN_POINT('',(43.,-3.18408167778311E-16,57.4));
#14154=CARTESIAN_POINT('',(58.,-3.18408167778311E-16,57.4));
#14155=CARTESIAN_POINT('',(43.,-2.59410389152015,59.825));
#14156=CARTESIAN_POINT('Origin',(43.,0.,60.));
#14157=CARTESIAN_POINT('',(43.,2.59410389152015,59.825));
#14158=CARTESIAN_POINT('Origin',(43.1166666666672,-9.08717545655691E-13,
60.0000000000008));
#14159=CARTESIAN_POINT('Origin',(43.,0.,60.));
#14160=CARTESIAN_POINT('Origin',(58.,36.,60.));
#14161=CARTESIAN_POINT('',(56.,36.,57.4));
#14162=CARTESIAN_POINT('Origin',(56.,36.,60.));
#14163=CARTESIAN_POINT('',(43.,36.,57.4));
#14164=CARTESIAN_POINT('',(58.,36.,57.4));
#14165=CARTESIAN_POINT('',(43.,33.4058961084799,59.825));
#14166=CARTESIAN_POINT('Origin',(43.,36.,60.));
#14167=CARTESIAN_POINT('',(43.,38.5941038915202,59.825));
#14168=CARTESIAN_POINT('Origin',(43.1166666666669,35.9999999999995,60.0000000000004));
#14169=CARTESIAN_POINT('Origin',(43.,36.,60.));
#14170=CARTESIAN_POINT('Origin',(-32.,97.,115.8875));
#14171=CARTESIAN_POINT('',(-32.,97.,118.3875));
#14172=CARTESIAN_POINT('Origin',(-32.,97.,115.8875));
#14173=CARTESIAN_POINT('',(-32.,82.,118.3875));
#14174=CARTESIAN_POINT('',(-32.,97.,118.3875));
#14175=CARTESIAN_POINT('Origin',(-32.,82.,115.8875));
#14176=CARTESIAN_POINT('Origin',(32.,97.,115.8875));
#14177=CARTESIAN_POINT('',(32.,97.,118.3875));
#14178=CARTESIAN_POINT('Origin',(32.,97.,115.8875));
#14179=CARTESIAN_POINT('',(32.,82.,118.3875));
#14180=CARTESIAN_POINT('',(32.,97.,118.3875));
#14181=CARTESIAN_POINT('Origin',(32.,82.,115.8875));
#14182=CARTESIAN_POINT('Origin',(0.,-86.,113.));
#14183=CARTESIAN_POINT('',(-1.11442858722409E-15,-87.,122.1));
#14184=CARTESIAN_POINT('Origin',(0.,-87.,113.));
#14185=CARTESIAN_POINT('',(-1.11442858722409E-15,-105.,122.1));
#14186=CARTESIAN_POINT('',(-1.11442858722409E-15,-86.,122.1));
#14187=CARTESIAN_POINT('Origin',(0.,-105.,113.));
#14188=CARTESIAN_POINT('Origin',(56.,49.,82.));
#14189=CARTESIAN_POINT('',(-22.,-87.,82.));
#14190=CARTESIAN_POINT('',(-22.,-105.,82.));
#14191=CARTESIAN_POINT('',(-22.,-87.,82.));
#14192=CARTESIAN_POINT('',(22.,-87.,82.));
#14193=CARTESIAN_POINT('',(-22.,-87.,82.));
#14194=CARTESIAN_POINT('',(22.,-105.,82.));
#14195=CARTESIAN_POINT('',(22.,-87.,82.));
#14196=CARTESIAN_POINT('',(56.,-105.,82.));
#14197=CARTESIAN_POINT('',(-56.,-105.,82.));
#14198=CARTESIAN_POINT('',(56.,105.,82.));
#14199=CARTESIAN_POINT('',(56.,49.,82.));
#14200=CARTESIAN_POINT('',(50.8,105.,82.));
#14201=CARTESIAN_POINT('',(-56.,105.,82.));
#14202=CARTESIAN_POINT('',(50.8,82.,82.));
#14203=CARTESIAN_POINT('',(50.8,105.,82.));
#14204=CARTESIAN_POINT('',(-50.8,82.,82.));
#14205=CARTESIAN_POINT('',(-50.8,82.,82.));
#14206=CARTESIAN_POINT('',(-50.8,105.,82.));
#14207=CARTESIAN_POINT('',(-50.8,105.,82.));
#14208=CARTESIAN_POINT('',(-56.,105.,82.));
#14209=CARTESIAN_POINT('',(-56.,105.,82.));
#14210=CARTESIAN_POINT('',(-56.,-105.,82.));
#14211=CARTESIAN_POINT('',(-56.,49.,82.));
#14212=CARTESIAN_POINT('',(-56.,-105.,82.));
#14213=CARTESIAN_POINT('',(8.,-79.,82.));
#14214=CARTESIAN_POINT('',(16.,-79.,82.));
#14215=CARTESIAN_POINT('',(56.,-79.,82.));
#14216=CARTESIAN_POINT('',(8.,-80.,82.));
#14217=CARTESIAN_POINT('',(8.,49.,82.));
#14218=CARTESIAN_POINT('',(-8.,-80.,82.));
#14219=CARTESIAN_POINT('',(56.,-80.,82.));
#14220=CARTESIAN_POINT('',(-8.,-79.,82.));
#14221=CARTESIAN_POINT('',(-8.,49.,82.));
#14222=CARTESIAN_POINT('',(-16.,-79.,82.));
#14223=CARTESIAN_POINT('',(56.,-79.,82.));
#14224=CARTESIAN_POINT('',(-16.,-47.,82.));
#14225=CARTESIAN_POINT('',(-16.,49.,82.));
#14226=CARTESIAN_POINT('',(-8.,-47.,82.));
#14227=CARTESIAN_POINT('',(56.,-47.,82.));
#14228=CARTESIAN_POINT('',(-8.,76.,82.));
#14229=CARTESIAN_POINT('',(-8.,49.,82.));
#14230=CARTESIAN_POINT('',(8.,76.,82.));
#14231=CARTESIAN_POINT('',(56.,76.,82.));
#14232=CARTESIAN_POINT('',(8.,-47.,82.));
#14233=CARTESIAN_POINT('',(8.,49.,82.));
#14234=CARTESIAN_POINT('',(16.,-47.,82.));
#14235=CARTESIAN_POINT('',(56.,-47.,82.));
#14236=CARTESIAN_POINT('',(16.,49.,82.));
#14237=CARTESIAN_POINT('Origin',(0.,-49.,0.));
#14238=CARTESIAN_POINT('',(16.,-49.,69.));
#14239=CARTESIAN_POINT('',(-16.,-49.,69.));
#14240=CARTESIAN_POINT('',(0.,-49.,69.));
#14241=CARTESIAN_POINT('',(-16.,-49.,70.));
#14242=CARTESIAN_POINT('',(-16.,-49.,0.));
#14243=CARTESIAN_POINT('',(-56.,-49.,70.));
#14244=CARTESIAN_POINT('',(0.,-49.,70.));
#14245=CARTESIAN_POINT('',(-56.,-49.,50.3));
#14246=CARTESIAN_POINT('',(-56.,-49.,82.));
#14247=CARTESIAN_POINT('',(-33.45,-49.,50.3));
#14248=CARTESIAN_POINT('',(-56.,-49.,50.3));
#14249=CARTESIAN_POINT('',(-45.45,-49.,68.3));
#14250=CARTESIAN_POINT('',(-33.45,-49.,50.3));
#14251=CARTESIAN_POINT('',(48.65,-49.,68.3));
#14252=CARTESIAN_POINT('',(-45.45,-49.,68.3));
#14253=CARTESIAN_POINT('',(36.65,-49.,50.3));
#14254=CARTESIAN_POINT('',(48.65,-49.,68.3));
#14255=CARTESIAN_POINT('',(56.,-49.,50.3));
#14256=CARTESIAN_POINT('',(36.65,-49.,50.3));
#14257=CARTESIAN_POINT('',(56.,-49.,70.));
#14258=CARTESIAN_POINT('',(56.,-49.,50.3));
#14259=CARTESIAN_POINT('',(16.,-49.,70.));
#14260=CARTESIAN_POINT('',(0.,-49.,70.));
#14261=CARTESIAN_POINT('',(16.,-49.,0.));
#14262=CARTESIAN_POINT('Origin',(0.,0.,70.));
#14263=CARTESIAN_POINT('',(-16.,-79.,70.));
#14264=CARTESIAN_POINT('',(-16.,0.,70.));
#14265=CARTESIAN_POINT('',(16.,-79.,70.));
#14266=CARTESIAN_POINT('',(0.,-79.,70.));
#14267=CARTESIAN_POINT('',(16.,0.,70.));
#14268=CARTESIAN_POINT('',(56.,-105.,70.));
#14269=CARTESIAN_POINT('',(56.,-105.,70.));
#14270=CARTESIAN_POINT('',(-56.,-105.,70.));
#14271=CARTESIAN_POINT('',(-56.,-105.,70.));
#14272=CARTESIAN_POINT('',(-56.,-105.,70.));
#14273=CARTESIAN_POINT('Origin',(8.,76.,78.));
#14274=CARTESIAN_POINT('',(8.,-79.,78.));
#14275=CARTESIAN_POINT('',(8.,-79.,78.));
#14276=CARTESIAN_POINT('',(8.,-80.,78.));
#14277=CARTESIAN_POINT('',(8.,76.,78.));
#14278=CARTESIAN_POINT('',(8.,-80.,78.));
#14279=CARTESIAN_POINT('Origin',(8.,76.,78.));
#14280=CARTESIAN_POINT('',(8.,76.,78.));
#14281=CARTESIAN_POINT('',(8.,-47.,78.));
#14282=CARTESIAN_POINT('',(8.,76.,78.));
#14283=CARTESIAN_POINT('',(8.,-47.,78.));
#14284=CARTESIAN_POINT('',(8.,76.,78.));
#14285=CARTESIAN_POINT('Origin',(-8.,76.,83.));
#14286=CARTESIAN_POINT('',(-8.,-79.,78.));
#14287=CARTESIAN_POINT('',(-8.,-80.,78.));
#14288=CARTESIAN_POINT('',(-8.,76.,78.));
#14289=CARTESIAN_POINT('',(-8.,-79.,83.));
#14290=CARTESIAN_POINT('',(-8.,-80.,83.));
#14291=CARTESIAN_POINT('Origin',(-8.,76.,83.));
#14292=CARTESIAN_POINT('',(-8.,-47.,78.));
#14293=CARTESIAN_POINT('',(-8.,-47.,83.));
#14294=CARTESIAN_POINT('',(-8.,76.,78.));
#14295=CARTESIAN_POINT('',(-8.,76.,78.));
#14296=CARTESIAN_POINT('',(-8.,76.,83.));
#14297=CARTESIAN_POINT('Origin',(16.,76.,78.));
#14298=CARTESIAN_POINT('',(16.,-79.,78.));
#14299=CARTESIAN_POINT('',(16.,-79.,78.));
#14300=CARTESIAN_POINT('',(16.,-80.,78.));
#14301=CARTESIAN_POINT('',(16.,76.,78.));
#14302=CARTESIAN_POINT('',(16.,-80.,78.));
#14303=CARTESIAN_POINT('Origin',(16.,76.,78.));
#14304=CARTESIAN_POINT('',(16.,76.,78.));
#14305=CARTESIAN_POINT('',(16.,-47.,78.));
#14306=CARTESIAN_POINT('',(16.,76.,78.));
#14307=CARTESIAN_POINT('',(16.,-47.,78.));
#14308=CARTESIAN_POINT('',(16.,76.,78.));
#14309=CARTESIAN_POINT('Origin',(-16.,76.,72.));
#14310=CARTESIAN_POINT('',(16.,-79.,72.));
#14311=CARTESIAN_POINT('',(16.,-80.,72.));
#14312=CARTESIAN_POINT('',(16.,76.,72.));
#14313=CARTESIAN_POINT('',(-16.,-79.,72.));
#14314=CARTESIAN_POINT('',(-16.,-79.,72.));
#14315=CARTESIAN_POINT('',(-16.,-80.,72.));
#14316=CARTESIAN_POINT('',(-16.,76.,72.));
#14317=CARTESIAN_POINT('',(-16.,-80.,72.));
#14318=CARTESIAN_POINT('Origin',(-16.,76.,72.));
#14319=CARTESIAN_POINT('',(-16.,76.,72.));
#14320=CARTESIAN_POINT('',(-16.,-47.,72.));
#14321=CARTESIAN_POINT('',(-16.,76.,72.));
#14322=CARTESIAN_POINT('',(16.,-47.,72.));
#14323=CARTESIAN_POINT('',(-16.,-47.,72.));
#14324=CARTESIAN_POINT('',(16.,76.,72.));
#14325=CARTESIAN_POINT('',(16.,76.,72.));
#14326=CARTESIAN_POINT('',(-16.,76.,72.));
#14327=CARTESIAN_POINT('Origin',(-8.,76.,78.));
#14328=CARTESIAN_POINT('',(-16.,-79.,78.));
#14329=CARTESIAN_POINT('',(-16.,-80.,78.));
#14330=CARTESIAN_POINT('',(-16.,76.,78.));
#14331=CARTESIAN_POINT('',(-8.,-79.,78.));
#14332=CARTESIAN_POINT('',(-8.,-80.,78.));
#14333=CARTESIAN_POINT('Origin',(-8.,76.,78.));
#14334=CARTESIAN_POINT('',(-16.,-47.,78.));
#14335=CARTESIAN_POINT('',(-8.,-47.,78.));
#14336=CARTESIAN_POINT('',(-16.,76.,78.));
#14337=CARTESIAN_POINT('',(-16.,76.,78.));
#14338=CARTESIAN_POINT('',(-8.,76.,78.));
#14339=CARTESIAN_POINT('Origin',(48.65,49.,68.3));
#14340=CARTESIAN_POINT('',(48.65,49.,68.3));
#14341=CARTESIAN_POINT('',(48.65,49.,68.3));
#14342=CARTESIAN_POINT('',(36.65,49.,50.3));
#14343=CARTESIAN_POINT('',(48.65,49.,68.3));
#14344=CARTESIAN_POINT('',(36.65,49.,50.3));
#14345=CARTESIAN_POINT('',(43.,49.,59.825));
#14346=CARTESIAN_POINT('',(43.,49.,59.825));
#14347=CARTESIAN_POINT('',(43.,49.,59.825));
#14348=CARTESIAN_POINT('Origin',(56.,49.,50.3));
#14349=CARTESIAN_POINT('',(56.,49.,70.));
#14350=CARTESIAN_POINT('',(56.,49.,50.3));
#14351=CARTESIAN_POINT('',(56.,49.,50.3));
#14352=CARTESIAN_POINT('',(56.,105.,70.));
#14353=CARTESIAN_POINT('',(56.,-105.,70.));
#14354=CARTESIAN_POINT('',(56.,105.,82.));
#14355=CARTESIAN_POINT('',(56.,-105.,82.));
#14356=CARTESIAN_POINT('',(56.,49.,50.3));
#14357=CARTESIAN_POINT('Origin',(36.65,49.,50.3));
#14358=CARTESIAN_POINT('',(36.65,49.,50.3));
#14359=CARTESIAN_POINT('Origin',(-45.45,49.,68.3));
#14360=CARTESIAN_POINT('',(-45.45,49.,68.3));
#14361=CARTESIAN_POINT('',(-45.45,49.,68.3));
#14362=CARTESIAN_POINT('',(-45.45,49.,68.3));
#14363=CARTESIAN_POINT('Origin',(-33.45,49.,50.3));
#14364=CARTESIAN_POINT('',(-33.45,49.,50.3));
#14365=CARTESIAN_POINT('',(-33.45,49.,50.3));
#14366=CARTESIAN_POINT('',(-33.45,49.,50.3));
#14367=CARTESIAN_POINT('Origin',(-56.,49.,50.3));
#14368=CARTESIAN_POINT('',(-56.,49.,50.3));
#14369=CARTESIAN_POINT('',(-56.,49.,50.3));
#14370=CARTESIAN_POINT('',(-56.,49.,50.3));
#14371=CARTESIAN_POINT('Origin',(-56.,49.,82.));
#14372=CARTESIAN_POINT('',(-56.,-105.,82.));
#14373=CARTESIAN_POINT('',(-56.,105.,70.));
#14374=CARTESIAN_POINT('',(-56.,105.,82.));
#14375=CARTESIAN_POINT('',(-56.,49.,70.));
#14376=CARTESIAN_POINT('',(-56.,-105.,70.));
#14377=CARTESIAN_POINT('',(-56.,49.,82.));
#14378=CARTESIAN_POINT('Origin',(0.,49.,0.));
#14379=CARTESIAN_POINT('',(0.,49.,70.));
#14380=CARTESIAN_POINT('Origin',(-56.,-105.,82.));
#14381=CARTESIAN_POINT('',(22.,-105.,119.));
#14382=CARTESIAN_POINT('',(22.,-105.,82.));
#14383=CARTESIAN_POINT('',(12.0000000000003,-105.,129.));
#14384=CARTESIAN_POINT('',(22.,-105.,119.));
#14385=CARTESIAN_POINT('',(-12.,-105.,129.));
#14386=CARTESIAN_POINT('',(12.0000000000003,-105.,129.));
#14387=CARTESIAN_POINT('',(-22.,-105.,119.000000000001));
#14388=CARTESIAN_POINT('',(-12.,-105.,129.));
#14389=CARTESIAN_POINT('',(-22.,-105.,119.000000000001));
#14390=CARTESIAN_POINT('Origin',(0.,0.,70.));
#14391=CARTESIAN_POINT('',(-56.,105.,70.));
#14392=CARTESIAN_POINT('Origin',(-56.,105.,82.));
#14393=CARTESIAN_POINT('',(-50.8,105.,127.35));
#14394=CARTESIAN_POINT('',(-50.8,105.,127.35));
#14395=CARTESIAN_POINT('',(-44.8,105.,133.35));
#14396=CARTESIAN_POINT('',(-44.8,105.,133.35));
#14397=CARTESIAN_POINT('',(44.8000000000001,105.,133.35));
#14398=CARTESIAN_POINT('',(44.8000000000001,105.,133.35));
#14399=CARTESIAN_POINT('',(50.8,105.,127.35));
#14400=CARTESIAN_POINT('',(50.8,105.,127.35));
#14401=CARTESIAN_POINT('',(50.8,105.,82.));
#14402=CARTESIAN_POINT('Origin',(-50.8,105.,127.35));
#14403=CARTESIAN_POINT('',(-50.8,82.,127.35));
#14404=CARTESIAN_POINT('',(-50.8,82.,127.35));
#14405=CARTESIAN_POINT('',(-50.8,105.,127.35));
#14406=CARTESIAN_POINT('Origin',(-44.8,105.,133.35));
#14407=CARTESIAN_POINT('',(-44.8,82.,133.35));
#14408=CARTESIAN_POINT('',(-44.8,82.,133.35));
#14409=CARTESIAN_POINT('',(-44.8,105.,133.35));
#14410=CARTESIAN_POINT('Origin',(44.8000000000001,105.,133.35));
#14411=CARTESIAN_POINT('',(44.8000000000001,82.,133.35));
#14412=CARTESIAN_POINT('',(44.8000000000001,82.,133.35));
#14413=CARTESIAN_POINT('',(44.8000000000001,105.,133.35));
#14414=CARTESIAN_POINT('Origin',(50.8,105.,127.35));
#14415=CARTESIAN_POINT('',(50.8,82.,127.35));
#14416=CARTESIAN_POINT('',(50.8,82.,127.35));
#14417=CARTESIAN_POINT('',(50.8,105.,127.35));
#14418=CARTESIAN_POINT('Origin',(50.8,105.,82.));
#14419=CARTESIAN_POINT('',(50.8,82.,82.));
#14420=CARTESIAN_POINT('Origin',(0.,82.,0.));
#14421=CARTESIAN_POINT('Origin',(-22.,-87.,119.000000000001));
#14422=CARTESIAN_POINT('',(-22.,-87.,119.000000000001));
#14423=CARTESIAN_POINT('',(-22.,-87.,119.000000000001));
#14424=CARTESIAN_POINT('',(-22.,-87.,119.000000000001));
#14425=CARTESIAN_POINT('Origin',(-12.,-87.,129.));
#14426=CARTESIAN_POINT('',(-12.,-87.,129.));
#14427=CARTESIAN_POINT('',(-12.,-87.,129.));
#14428=CARTESIAN_POINT('',(-12.,-87.,129.));
#14429=CARTESIAN_POINT('Origin',(12.0000000000003,-87.,129.));
#14430=CARTESIAN_POINT('',(12.0000000000003,-87.,129.));
#14431=CARTESIAN_POINT('',(12.0000000000003,-87.,129.));
#14432=CARTESIAN_POINT('',(12.0000000000003,-87.,129.));
#14433=CARTESIAN_POINT('Origin',(22.,-87.,119.));
#14434=CARTESIAN_POINT('',(22.,-87.,119.));
#14435=CARTESIAN_POINT('',(22.,-87.,119.));
#14436=CARTESIAN_POINT('',(22.,-87.,119.));
#14437=CARTESIAN_POINT('Origin',(22.,-87.,82.));
#14438=CARTESIAN_POINT('',(22.,-87.,82.));
#14439=CARTESIAN_POINT('Origin',(0.,-87.,0.));
#14440=CARTESIAN_POINT('Origin',(0.,76.,0.));
#14441=CARTESIAN_POINT('',(-16.,76.,78.));
#14442=CARTESIAN_POINT('',(16.,76.,72.));
#14443=CARTESIAN_POINT('Origin',(0.,-80.,0.));
#14444=CARTESIAN_POINT('',(16.,-80.,72.));
#14445=CARTESIAN_POINT('',(-16.,-80.,78.));
#14446=CARTESIAN_POINT('Origin',(16.,76.,72.));
#14447=CARTESIAN_POINT('',(16.,-79.,83.));
#14448=CARTESIAN_POINT('',(16.,-79.,83.));
#14449=CARTESIAN_POINT('',(16.,-47.,83.));
#14450=CARTESIAN_POINT('',(16.,-47.,69.));
#14451=CARTESIAN_POINT('',(16.,-47.,83.));
#14452=CARTESIAN_POINT('',(16.,-79.,69.));
#14453=CARTESIAN_POINT('Origin',(-16.,76.,78.));
#14454=CARTESIAN_POINT('',(-16.,-79.,83.));
#14455=CARTESIAN_POINT('',(-16.,-79.,83.));
#14456=CARTESIAN_POINT('',(-16.,-47.,69.));
#14457=CARTESIAN_POINT('',(-16.,-47.,69.));
#14458=CARTESIAN_POINT('',(-16.,-47.,83.));
#14459=CARTESIAN_POINT('',(-16.,-47.,83.));
#14460=CARTESIAN_POINT('Origin',(32.,97.,115.8875));
#14461=CARTESIAN_POINT('Origin',(-32.,97.,115.8875));
#14462=CARTESIAN_POINT('Origin',(43.,36.,60.));
#14463=CARTESIAN_POINT('Origin',(43.,0.,60.));
#14464=CARTESIAN_POINT('Origin',(43.,-36.,60.));
#14465=CARTESIAN_POINT('Origin',(-16.,-79.,83.));
#14466=CARTESIAN_POINT('Origin',(16.,-47.,83.));
#14467=CARTESIAN_POINT('Origin',(16.,-47.,83.));
#14468=CARTESIAN_POINT('',(16.,-47.,69.));
#14469=CARTESIAN_POINT('Origin',(-16.,-79.,83.));
#14470=CARTESIAN_POINT('Origin',(0.,0.,69.));
#14471=CARTESIAN_POINT('Origin',(-16.,-79.,83.));
#14472=CARTESIAN_POINT('Origin',(16.,-47.,83.));
#16550=UNCERTAINTY_MEASURE_WITH_UNIT(LENGTH_MEASURE(0.01),#16599,
'DISTANCE_ACCURACY_VALUE',
'Maximum model space distance between geometric entities at asserted c
onnectivities');
#16572=UNCERTAINTY_MEASURE_WITH_UNIT(LENGTH_MEASURE(0.01),#16599,
'DISTANCE_ACCURACY_VALUE',
'Maximum model space distance between geometric entities at asserted c
onnectivities');
#16576=(
GEOMETRIC_REPRESENTATION_CONTEXT(3)
GLOBAL_UNCERTAINTY_ASSIGNED_CONTEXT((#16550))
GLOBAL_UNIT_ASSIGNED_CONTEXT((#16599,#16601,#16602))
REPRESENTATION_CONTEXT('','3D')
);
#16598=(
GEOMETRIC_REPRESENTATION_CONTEXT(3)
GLOBAL_UNCERTAINTY_ASSIGNED_CONTEXT((#16572))
GLOBAL_UNIT_ASSIGNED_CONTEXT((#16599,#16601,#16602))
REPRESENTATION_CONTEXT('','3D')
);
#16599=(
LENGTH_UNIT()
NAMED_UNIT(*)
SI_UNIT(.MILLI.,.METRE.)
);
#16601=(
NAMED_UNIT(*)
PLANE_ANGLE_UNIT()
SI_UNIT($,.RADIAN.)
);
#16602=(
NAMED_UNIT(*)
SI_UNIT($,.STERADIAN.)
SOLID_ANGLE_UNIT()
);
#16606=SHAPE_DEFINITION_REPRESENTATION(#16631,#16700);
#16631=PRODUCT_DEFINITION_SHAPE('',$,#16726);
#16700=SHAPE_REPRESENTATION('',(#10189),#16576);
#16722=PRODUCT_DEFINITION_CONTEXT('part definition',#16799,'design');
#16726=PRODUCT_DEFINITION('P03_Upper_Vise_Body','P03_Upper_Vise_Body',#16751,
#16722);
#16751=PRODUCT_DEFINITION_FORMATION('',$,#16804);
#16799=APPLICATION_CONTEXT(
'Core Data for Automotive Mechanical Design Process');
#16800=PRODUCT_CONTEXT('part definition',#16799,'mechanical');
#16804=PRODUCT('P03_Upper_Vise_Body','P03_Upper_Vise_Body',$,(#16800));
#16830=PRESENTATION_STYLE_ASSIGNMENT((#16839));
#16839=SURFACE_STYLE_USAGE(.BOTH.,#16848);
#16848=SURFACE_SIDE_STYLE('',(#16857));
#16857=SURFACE_STYLE_FILL_AREA(#16866);
#16866=FILL_AREA_STYLE('Dark Blue',(#16875));
#16875=FILL_AREA_STYLE_COLOUR('Dark Blue',#16884);
#16884=COLOUR_RGB('Dark Blue',0.,0.125490196078431,0.376470588235294);
ENDSEC;
END-ISO-10303-21;
